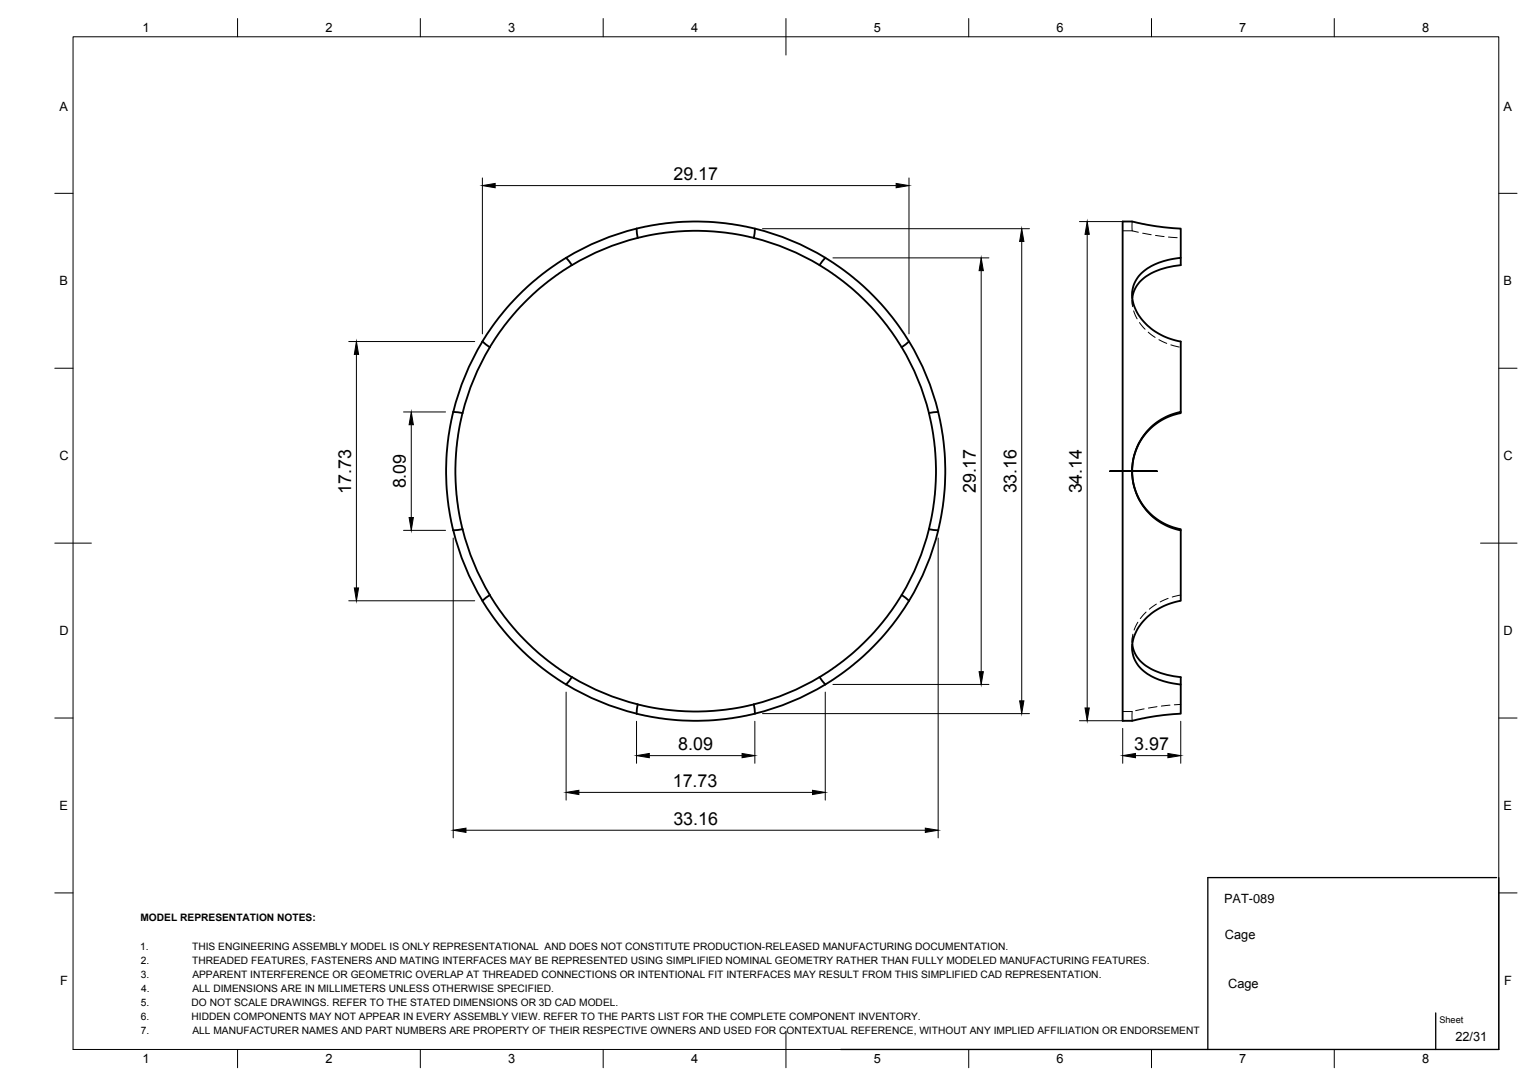
ISO-10303-21;
HEADER;
/* Generated by software containing ST-Developer
 * from STEP Tools, Inc. (www.steptools.com) 
 */

FILE_DESCRIPTION(
/* description */ ('Rotary union on bearing shaft'),
/* implementation_level */ '2;1');

FILE_NAME(
/* name */ 'Cage.step',
/* time_stamp */ '2026-10-28T03:24:01-07:00',
/* author */ (''),
/* organization */ (''),
/* preprocessor_version */ 'ST-DEVELOPER v20.2',
/* originating_system */ 'Autodesk Translation Framework v15.17.0.0',
/* authorisation */ '');

FILE_SCHEMA (('AUTOMOTIVE_DESIGN { 1 0 10303 214 3 1 1 }'));
ENDSEC;

DATA;
#10=MECHANICAL_DESIGN_GEOMETRIC_PRESENTATION_REPRESENTATION('',(#334),#9448);
#193=SPHERICAL_SURFACE('',#5486,0.412776);
#194=SPHERICAL_SURFACE('',#5502,0.412776);
#195=SPHERICAL_SURFACE('',#5507,0.412776);
#196=SPHERICAL_SURFACE('',#5512,0.412776);
#197=SPHERICAL_SURFACE('',#5517,0.412776);
#198=SPHERICAL_SURFACE('',#5522,0.412776);
#199=SPHERICAL_SURFACE('',#5527,0.412776);
#200=SPHERICAL_SURFACE('',#5535,0.412776);
#233=B_SPLINE_CURVE_WITH_KNOTS('',3,(#8136,#8137,#8138,#8139,#8140,#8141,
#8142,#8143,#8144,#8145,#8146,#8147,#8148,#8149,#8150,#8151,#8152,#8153,
#8154,#8155,#8156,#8157),.UNSPECIFIED.,.F.,.F.,(4,2,2,2,2,2,2,2,2,2,4),
(0.0789094028588958,0.210573405340968,0.315860108011452,0.421146810681936,
0.522142632548711,0.623138454415485,0.72413427628226,0.825130098149035,
0.930416800819519,1.03570350349,1.16736750597208),.UNSPECIFIED.);
#234=B_SPLINE_CURVE_WITH_KNOTS('',3,(#8161,#8162,#8163,#8164,#8165,#8166,
#8167,#8168,#8169,#8170,#8171,#8172,#8173,#8174,#8175,#8176,#8177,#8178,
#8179,#8180,#8181,#8182),.UNSPECIFIED.,.F.,.F.,(4,2,2,2,2,2,2,2,2,2,4),
(0.0774793363974613,0.142088896491891,0.284177792983782,0.411119756996526,
0.514392970548519,0.617666184100513,0.720939397652506,0.8242126112045,0.951154575217244,
1.09324347170913,1.15785303180356),.UNSPECIFIED.);
#235=B_SPLINE_CURVE_WITH_KNOTS('',3,(#8188,#8189,#8190,#8191,#8192,#8193,
#8194,#8195,#8196,#8197,#8198,#8199,#8200,#8201,#8202,#8203,#8204,#8205,
#8206,#8207,#8208,#8209),.UNSPECIFIED.,.F.,.F.,(4,2,2,2,2,2,2,2,2,2,4),
(0.0774793363974613,0.142088896491891,0.284177792983782,0.411119756996525,
0.514392970548519,0.617666184100513,0.720939397652506,0.8242126112045,0.951154575217243,
1.09324347170913,1.15785303180356),.UNSPECIFIED.);
#236=B_SPLINE_CURVE_WITH_KNOTS('',3,(#8213,#8214,#8215,#8216,#8217,#8218,
#8219,#8220,#8221,#8222,#8223,#8224,#8225,#8226,#8227,#8228,#8229,#8230,
#8231,#8232,#8233,#8234),.UNSPECIFIED.,.F.,.F.,(4,2,2,2,2,2,2,2,2,2,4),
(0.0774793363974614,0.142088896491891,0.284177792983781,0.411119756996525,
0.514392970548519,0.617666184100512,0.720939397652506,0.824212611204499,
0.951154575217243,1.09324347170913,1.15785303180356),.UNSPECIFIED.);
#237=B_SPLINE_CURVE_WITH_KNOTS('',3,(#8238,#8239,#8240,#8241,#8242,#8243,
#8244,#8245,#8246,#8247,#8248,#8249),.UNSPECIFIED.,.F.,.F.,(4,2,2,2,2,4),
(0.0774793363974613,0.142088896491891,0.284177792983781,0.411119756996525,
0.514392970548519,0.617666184100512),.UNSPECIFIED.);
#238=B_SPLINE_CURVE_WITH_KNOTS('',3,(#8254,#8255,#8256,#8257,#8258,#8259,
#8260,#8261,#8262,#8263,#8264,#8265),.UNSPECIFIED.,.F.,.F.,(4,2,2,2,2,4),
(0.617666184100512,0.720939397652506,0.824212611204499,0.951154575217243,
1.09324347170913,1.15785303180356),.UNSPECIFIED.);
#239=B_SPLINE_CURVE_WITH_KNOTS('',3,(#8269,#8270,#8271,#8272,#8273,#8274,
#8275,#8276,#8277,#8278,#8279,#8280,#8281,#8282,#8283,#8284,#8285,#8286,
#8287,#8288,#8289,#8290),.UNSPECIFIED.,.F.,.F.,(4,2,2,2,2,2,2,2,2,2,4),
(0.0774793363974613,0.142088896491891,0.284177792983782,0.411119756996526,
0.514392970548519,0.617666184100513,0.720939397652507,0.8242126112045,0.951154575217245,
1.09324347170914,1.15785303180356),.UNSPECIFIED.);
#240=B_SPLINE_CURVE_WITH_KNOTS('',3,(#8294,#8295,#8296,#8297,#8298,#8299,
#8300,#8301,#8302,#8303,#8304,#8305,#8306,#8307,#8308,#8309,#8310,#8311,
#8312,#8313,#8314,#8315),.UNSPECIFIED.,.F.,.F.,(4,2,2,2,2,2,2,2,2,2,4),
(0.0774793363974613,0.142088896491891,0.284177792983782,0.411119756996526,
0.514392970548519,0.617666184100513,0.720939397652506,0.824212611204499,
0.951154575217243,1.09324347170913,1.15785303180356),.UNSPECIFIED.);
#241=B_SPLINE_CURVE_WITH_KNOTS('',3,(#8319,#8320,#8321,#8322,#8323,#8324,
#8325,#8326,#8327,#8328,#8329,#8330,#8331,#8332,#8333,#8334,#8335,#8336,
#8337,#8338,#8339,#8340),.UNSPECIFIED.,.F.,.F.,(4,2,2,2,2,2,2,2,2,2,4),
(0.0774793363974613,0.142088896491891,0.284177792983782,0.411119756996526,
0.514392970548519,0.617666184100513,0.720939397652506,0.8242126112045,0.951154575217244,
1.09324347170913,1.15785303180356),.UNSPECIFIED.);
#242=B_SPLINE_CURVE_WITH_KNOTS('',3,(#8344,#8345,#8346,#8347,#8348,#8349,
#8350,#8351,#8352,#8353,#8354,#8355,#8356,#8357,#8358,#8359,#8360,#8361,
#8362,#8363,#8364,#8365),.UNSPECIFIED.,.F.,.F.,(4,2,2,2,2,2,2,2,2,2,4),
(0.0774793363974613,0.142088896491891,0.284177792983782,0.411119756996526,
0.514392970548519,0.617666184100513,0.720939397652506,0.8242126112045,0.951154575217243,
1.09324347170913,1.15785303180356),.UNSPECIFIED.);
#243=B_SPLINE_CURVE_WITH_KNOTS('',3,(#8373,#8374,#8375,#8376,#8377,#8378,
#8379,#8380,#8381,#8382,#8383,#8384,#8385,#8386,#8387,#8388,#8389,#8390,
#8391,#8392,#8393,#8394),.UNSPECIFIED.,.F.,.F.,(4,2,2,2,2,2,2,2,2,2,4),
(0.0789094028588958,0.210573405340968,0.315860108011452,0.421146810681936,
0.522142632548711,0.623138454415485,0.72413427628226,0.825130098149035,
0.930416800819519,1.03570350349,1.16736750597208),.UNSPECIFIED.);
#244=B_SPLINE_CURVE_WITH_KNOTS('',3,(#8402,#8403,#8404,#8405,#8406,#8407,
#8408,#8409,#8410,#8411,#8412,#8413,#8414,#8415,#8416,#8417,#8418,#8419,
#8420,#8421,#8422,#8423),.UNSPECIFIED.,.F.,.F.,(4,2,2,2,2,2,2,2,2,2,4),
(0.0789094028588958,0.210573405340969,0.315860108011453,0.421146810681937,
0.522142632548712,0.623138454415486,0.724134276282261,0.825130098149035,
0.930416800819519,1.03570350349,1.16736750597208),.UNSPECIFIED.);
#245=B_SPLINE_CURVE_WITH_KNOTS('',3,(#8432,#8433,#8434,#8435,#8436,#8437,
#8438,#8439,#8440,#8441,#8442,#8443),.UNSPECIFIED.,.F.,.F.,(4,2,2,2,2,4),
(0.0789094028588958,0.210573405340968,0.315860108011452,0.421146810681937,
0.522142632548711,0.623138454415486),.UNSPECIFIED.);
#246=B_SPLINE_CURVE_WITH_KNOTS('',3,(#8445,#8446,#8447,#8448,#8449,#8450,
#8451,#8452,#8453,#8454,#8455,#8456),.UNSPECIFIED.,.F.,.F.,(4,2,2,2,2,4),
(0.623138454415486,0.72413427628226,0.825130098149035,0.930416800819519,
1.03570350349,1.16736750597208),.UNSPECIFIED.);
#247=B_SPLINE_CURVE_WITH_KNOTS('',3,(#8463,#8464,#8465,#8466,#8467,#8468,
#8469,#8470,#8471,#8472,#8473,#8474,#8475,#8476,#8477,#8478,#8479,#8480,
#8481,#8482,#8483,#8484),.UNSPECIFIED.,.F.,.F.,(4,2,2,2,2,2,2,2,2,2,4),
(0.0789094028588958,0.210573405340968,0.315860108011452,0.421146810681936,
0.522142632548711,0.623138454415486,0.72413427628226,0.825130098149035,
0.930416800819519,1.03570350349,1.16736750597208),.UNSPECIFIED.);
#248=B_SPLINE_CURVE_WITH_KNOTS('',3,(#8492,#8493,#8494,#8495,#8496,#8497,
#8498,#8499,#8500,#8501,#8502,#8503,#8504,#8505,#8506,#8507,#8508,#8509,
#8510,#8511,#8512,#8513),.UNSPECIFIED.,.F.,.F.,(4,2,2,2,2,2,2,2,2,2,4),
(0.0789094028588957,0.210573405340968,0.315860108011452,0.421146810681936,
0.522142632548711,0.623138454415485,0.72413427628226,0.825130098149035,
0.930416800819519,1.03570350349,1.16736750597207),.UNSPECIFIED.);
#249=B_SPLINE_CURVE_WITH_KNOTS('',3,(#8521,#8522,#8523,#8524,#8525,#8526,
#8527,#8528,#8529,#8530,#8531,#8532,#8533,#8534,#8535,#8536,#8537,#8538,
#8539,#8540,#8541,#8542),.UNSPECIFIED.,.F.,.F.,(4,2,2,2,2,2,2,2,2,2,4),
(0.0789094028588958,0.210573405340968,0.315860108011452,0.421146810681936,
0.522142632548711,0.623138454415486,0.72413427628226,0.825130098149035,
0.930416800819519,1.03570350349,1.16736750597208),.UNSPECIFIED.);
#250=B_SPLINE_CURVE_WITH_KNOTS('',3,(#8551,#8552,#8553,#8554,#8555,#8556,
#8557,#8558,#8559,#8560,#8561,#8562,#8563,#8564,#8565,#8566,#8567,#8568,
#8569,#8570,#8571,#8572),.UNSPECIFIED.,.F.,.F.,(4,2,2,2,2,2,2,2,2,2,4),
(0.0789094028588958,0.210573405340968,0.315860108011452,0.421146810681936,
0.522142632548711,0.623138454415485,0.72413427628226,0.825130098149035,
0.930416800819519,1.03570350349,1.16736750597208),.UNSPECIFIED.);
#273=SHAPE_REPRESENTATION_RELATIONSHIP('SRR','None',#9574,#300);
#300=ADVANCED_BREP_SHAPE_REPRESENTATION('',(#369),#9434);
#334=STYLED_ITEM('',(#9778),#369);
#369=MANIFOLD_SOLID_BREP('Continuous crown cage',#4889);
#448=FACE_BOUND('',#1176,.T.);
#554=PLANE('',#5499);
#555=PLANE('',#5504);
#556=PLANE('',#5509);
#557=PLANE('',#5514);
#558=PLANE('',#5519);
#559=PLANE('',#5524);
#560=PLANE('',#5533);
#561=PLANE('',#5537);
#562=PLANE('',#5538);
#791=FACE_OUTER_BOUND('',#1158,.T.);
#792=FACE_OUTER_BOUND('',#1159,.T.);
#793=FACE_OUTER_BOUND('',#1160,.T.);
#794=FACE_OUTER_BOUND('',#1161,.T.);
#795=FACE_OUTER_BOUND('',#1162,.T.);
#796=FACE_OUTER_BOUND('',#1163,.T.);
#797=FACE_OUTER_BOUND('',#1164,.T.);
#798=FACE_OUTER_BOUND('',#1165,.T.);
#799=FACE_OUTER_BOUND('',#1166,.T.);
#800=FACE_OUTER_BOUND('',#1167,.T.);
#801=FACE_OUTER_BOUND('',#1168,.T.);
#802=FACE_OUTER_BOUND('',#1169,.T.);
#803=FACE_OUTER_BOUND('',#1170,.T.);
#804=FACE_OUTER_BOUND('',#1171,.T.);
#805=FACE_OUTER_BOUND('',#1172,.T.);
#806=FACE_OUTER_BOUND('',#1173,.T.);
#807=FACE_OUTER_BOUND('',#1174,.T.);
#808=FACE_OUTER_BOUND('',#1175,.T.);
#809=FACE_OUTER_BOUND('',#1177,.T.);
#1158=EDGE_LOOP('',(#3803,#3804,#3805,#3806));
#1159=EDGE_LOOP('',(#3807,#3808,#3809,#3810,#3811,#3812,#3813,#3814,#3815,
#3816,#3817,#3818,#3819,#3820,#3821,#3822,#3823,#3824,#3825,#3826));
#1160=EDGE_LOOP('',(#3827,#3828,#3829,#3830));
#1161=EDGE_LOOP('',(#3831,#3832,#3833,#3834));
#1162=EDGE_LOOP('',(#3835,#3836,#3837,#3838));
#1163=EDGE_LOOP('',(#3839,#3840,#3841,#3842));
#1164=EDGE_LOOP('',(#3843,#3844,#3845,#3846));
#1165=EDGE_LOOP('',(#3847,#3848,#3849,#3850,#3851,#3852));
#1166=EDGE_LOOP('',(#3853,#3854,#3855,#3856));
#1167=EDGE_LOOP('',(#3857,#3858,#3859,#3860));
#1168=EDGE_LOOP('',(#3861,#3862,#3863,#3864));
#1169=EDGE_LOOP('',(#3865,#3866,#3867,#3868));
#1170=EDGE_LOOP('',(#3869,#3870,#3871,#3872));
#1171=EDGE_LOOP('',(#3873,#3874,#3875,#3876));
#1172=EDGE_LOOP('',(#3877,#3878,#3879,#3880,#3881,#3882,#3883,#3884,#3885,
#3886,#3887,#3888,#3889,#3890,#3891,#3892,#3893,#3894,#3895,#3896));
#1173=EDGE_LOOP('',(#3897,#3898,#3899,#3900));
#1174=EDGE_LOOP('',(#3901,#3902,#3903,#3904));
#1175=EDGE_LOOP('',(#3905));
#1176=EDGE_LOOP('',(#3906));
#1177=EDGE_LOOP('',(#3907,#3908,#3909,#3910));
#1492=LINE('',#8251,#1812);
#1493=LINE('',#8547,#1813);
#1812=VECTOR('',#6537,1.706752);
#1813=VECTOR('',#6614,1.643248);
#2130=CIRCLE('',#5487,0.405071403305639);
#2131=CIRCLE('',#5488,0.405071403305639);
#2132=CIRCLE('',#5490,1.706752);
#2133=CIRCLE('',#5491,1.706752);
#2134=CIRCLE('',#5492,1.706752);
#2135=CIRCLE('',#5493,1.706752);
#2136=CIRCLE('',#5494,1.706752);
#2137=CIRCLE('',#5495,1.706752);
#2138=CIRCLE('',#5496,1.706752);
#2139=CIRCLE('',#5497,1.706752);
#2140=CIRCLE('',#5498,1.706752);
#2141=CIRCLE('',#5500,1.643248);
#2142=CIRCLE('',#5501,0.405071403305639);
#2143=CIRCLE('',#5503,0.405071403305639);
#2144=CIRCLE('',#5505,1.643248);
#2145=CIRCLE('',#5506,0.405071403305639);
#2146=CIRCLE('',#5508,0.405071403305639);
#2147=CIRCLE('',#5510,1.643248);
#2148=CIRCLE('',#5511,0.405071403305639);
#2149=CIRCLE('',#5513,0.405071403305639);
#2150=CIRCLE('',#5515,1.643248);
#2151=CIRCLE('',#5516,0.405071403305639);
#2152=CIRCLE('',#5518,0.405071403305639);
#2153=CIRCLE('',#5520,1.643248);
#2154=CIRCLE('',#5521,0.405071403305639);
#2155=CIRCLE('',#5523,0.405071403305639);
#2156=CIRCLE('',#5525,1.643248);
#2157=CIRCLE('',#5526,0.405071403305639);
#2158=CIRCLE('',#5528,0.405071403305639);
#2159=CIRCLE('',#5530,1.643248);
#2160=CIRCLE('',#5531,1.643248);
#2161=CIRCLE('',#5532,1.643248);
#2162=CIRCLE('',#5534,0.405071403305639);
#2163=CIRCLE('',#5536,0.405071403305639);
#2440=VERTEX_POINT('',#8134);
#2441=VERTEX_POINT('',#8135);
#2442=VERTEX_POINT('',#8158);
#2443=VERTEX_POINT('',#8160);
#2444=VERTEX_POINT('',#8185);
#2445=VERTEX_POINT('',#8187);
#2446=VERTEX_POINT('',#8210);
#2447=VERTEX_POINT('',#8212);
#2448=VERTEX_POINT('',#8235);
#2449=VERTEX_POINT('',#8237);
#2450=VERTEX_POINT('',#8250);
#2451=VERTEX_POINT('',#8253);
#2452=VERTEX_POINT('',#8266);
#2453=VERTEX_POINT('',#8268);
#2454=VERTEX_POINT('',#8291);
#2455=VERTEX_POINT('',#8293);
#2456=VERTEX_POINT('',#8316);
#2457=VERTEX_POINT('',#8318);
#2458=VERTEX_POINT('',#8341);
#2459=VERTEX_POINT('',#8343);
#2460=VERTEX_POINT('',#8368);
#2461=VERTEX_POINT('',#8372);
#2462=VERTEX_POINT('',#8397);
#2463=VERTEX_POINT('',#8401);
#2464=VERTEX_POINT('',#8426);
#2465=VERTEX_POINT('',#8430);
#2466=VERTEX_POINT('',#8431);
#2467=VERTEX_POINT('',#8458);
#2468=VERTEX_POINT('',#8462);
#2469=VERTEX_POINT('',#8487);
#2470=VERTEX_POINT('',#8491);
#2471=VERTEX_POINT('',#8516);
#2472=VERTEX_POINT('',#8520);
#2473=VERTEX_POINT('',#8545);
#2474=VERTEX_POINT('',#8548);
#2475=VERTEX_POINT('',#8550);
#2929=EDGE_CURVE('',#2440,#2441,#233,.T.);
#2930=EDGE_CURVE('',#2442,#2440,#2130,.T.);
#2931=EDGE_CURVE('',#2443,#2442,#234,.T.);
#2932=EDGE_CURVE('',#2441,#2443,#2131,.T.);
#2933=EDGE_CURVE('',#2444,#2442,#2132,.T.);
#2934=EDGE_CURVE('',#2444,#2445,#235,.T.);
#2935=EDGE_CURVE('',#2446,#2445,#2133,.T.);
#2936=EDGE_CURVE('',#2446,#2447,#236,.T.);
#2937=EDGE_CURVE('',#2448,#2447,#2134,.T.);
#2938=EDGE_CURVE('',#2448,#2449,#237,.T.);
#2939=EDGE_CURVE('',#2449,#2450,#1492,.T.);
#2940=EDGE_CURVE('',#2450,#2450,#2135,.T.);
#2941=EDGE_CURVE('',#2449,#2451,#238,.T.);
#2942=EDGE_CURVE('',#2452,#2451,#2136,.T.);
#2943=EDGE_CURVE('',#2452,#2453,#239,.T.);
#2944=EDGE_CURVE('',#2454,#2453,#2137,.T.);
#2945=EDGE_CURVE('',#2454,#2455,#240,.T.);
#2946=EDGE_CURVE('',#2456,#2455,#2138,.T.);
#2947=EDGE_CURVE('',#2456,#2457,#241,.T.);
#2948=EDGE_CURVE('',#2458,#2457,#2139,.T.);
#2949=EDGE_CURVE('',#2458,#2459,#242,.T.);
#2950=EDGE_CURVE('',#2443,#2459,#2140,.T.);
#2951=EDGE_CURVE('',#2440,#2460,#2141,.T.);
#2952=EDGE_CURVE('',#2460,#2444,#2142,.T.);
#2953=EDGE_CURVE('',#2461,#2460,#243,.T.);
#2954=EDGE_CURVE('',#2445,#2461,#2143,.T.);
#2955=EDGE_CURVE('',#2461,#2462,#2144,.T.);
#2956=EDGE_CURVE('',#2462,#2446,#2145,.T.);
#2957=EDGE_CURVE('',#2463,#2462,#244,.T.);
#2958=EDGE_CURVE('',#2447,#2463,#2146,.T.);
#2959=EDGE_CURVE('',#2463,#2464,#2147,.T.);
#2960=EDGE_CURVE('',#2464,#2448,#2148,.T.);
#2961=EDGE_CURVE('',#2465,#2466,#245,.T.);
#2962=EDGE_CURVE('',#2451,#2465,#2149,.T.);
#2963=EDGE_CURVE('',#2466,#2464,#246,.T.);
#2964=EDGE_CURVE('',#2465,#2467,#2150,.T.);
#2965=EDGE_CURVE('',#2467,#2452,#2151,.T.);
#2966=EDGE_CURVE('',#2468,#2467,#247,.T.);
#2967=EDGE_CURVE('',#2453,#2468,#2152,.T.);
#2968=EDGE_CURVE('',#2468,#2469,#2153,.T.);
#2969=EDGE_CURVE('',#2469,#2454,#2154,.T.);
#2970=EDGE_CURVE('',#2470,#2469,#248,.T.);
#2971=EDGE_CURVE('',#2455,#2470,#2155,.T.);
#2972=EDGE_CURVE('',#2470,#2471,#2156,.T.);
#2973=EDGE_CURVE('',#2471,#2456,#2157,.T.);
#2974=EDGE_CURVE('',#2472,#2471,#249,.T.);
#2975=EDGE_CURVE('',#2457,#2472,#2158,.T.);
#2976=EDGE_CURVE('',#2473,#2473,#2159,.T.);
#2977=EDGE_CURVE('',#2473,#2466,#1493,.T.);
#2978=EDGE_CURVE('',#2474,#2441,#2160,.T.);
#2979=EDGE_CURVE('',#2474,#2475,#250,.T.);
#2980=EDGE_CURVE('',#2472,#2475,#2161,.T.);
#2981=EDGE_CURVE('',#2459,#2474,#2162,.T.);
#2982=EDGE_CURVE('',#2475,#2458,#2163,.T.);
#3803=ORIENTED_EDGE('',*,*,#2929,.F.);
#3804=ORIENTED_EDGE('',*,*,#2930,.F.);
#3805=ORIENTED_EDGE('',*,*,#2931,.F.);
#3806=ORIENTED_EDGE('',*,*,#2932,.F.);
#3807=ORIENTED_EDGE('',*,*,#2931,.T.);
#3808=ORIENTED_EDGE('',*,*,#2933,.F.);
#3809=ORIENTED_EDGE('',*,*,#2934,.T.);
#3810=ORIENTED_EDGE('',*,*,#2935,.F.);
#3811=ORIENTED_EDGE('',*,*,#2936,.T.);
#3812=ORIENTED_EDGE('',*,*,#2937,.F.);
#3813=ORIENTED_EDGE('',*,*,#2938,.T.);
#3814=ORIENTED_EDGE('',*,*,#2939,.T.);
#3815=ORIENTED_EDGE('',*,*,#2940,.F.);
#3816=ORIENTED_EDGE('',*,*,#2939,.F.);
#3817=ORIENTED_EDGE('',*,*,#2941,.T.);
#3818=ORIENTED_EDGE('',*,*,#2942,.F.);
#3819=ORIENTED_EDGE('',*,*,#2943,.T.);
#3820=ORIENTED_EDGE('',*,*,#2944,.F.);
#3821=ORIENTED_EDGE('',*,*,#2945,.T.);
#3822=ORIENTED_EDGE('',*,*,#2946,.F.);
#3823=ORIENTED_EDGE('',*,*,#2947,.T.);
#3824=ORIENTED_EDGE('',*,*,#2948,.F.);
#3825=ORIENTED_EDGE('',*,*,#2949,.T.);
#3826=ORIENTED_EDGE('',*,*,#2950,.F.);
#3827=ORIENTED_EDGE('',*,*,#2930,.T.);
#3828=ORIENTED_EDGE('',*,*,#2951,.T.);
#3829=ORIENTED_EDGE('',*,*,#2952,.T.);
#3830=ORIENTED_EDGE('',*,*,#2933,.T.);
#3831=ORIENTED_EDGE('',*,*,#2953,.F.);
#3832=ORIENTED_EDGE('',*,*,#2954,.F.);
#3833=ORIENTED_EDGE('',*,*,#2934,.F.);
#3834=ORIENTED_EDGE('',*,*,#2952,.F.);
#3835=ORIENTED_EDGE('',*,*,#2954,.T.);
#3836=ORIENTED_EDGE('',*,*,#2955,.T.);
#3837=ORIENTED_EDGE('',*,*,#2956,.T.);
#3838=ORIENTED_EDGE('',*,*,#2935,.T.);
#3839=ORIENTED_EDGE('',*,*,#2957,.F.);
#3840=ORIENTED_EDGE('',*,*,#2958,.F.);
#3841=ORIENTED_EDGE('',*,*,#2936,.F.);
#3842=ORIENTED_EDGE('',*,*,#2956,.F.);
#3843=ORIENTED_EDGE('',*,*,#2958,.T.);
#3844=ORIENTED_EDGE('',*,*,#2959,.T.);
#3845=ORIENTED_EDGE('',*,*,#2960,.T.);
#3846=ORIENTED_EDGE('',*,*,#2937,.T.);
#3847=ORIENTED_EDGE('',*,*,#2961,.F.);
#3848=ORIENTED_EDGE('',*,*,#2962,.F.);
#3849=ORIENTED_EDGE('',*,*,#2941,.F.);
#3850=ORIENTED_EDGE('',*,*,#2938,.F.);
#3851=ORIENTED_EDGE('',*,*,#2960,.F.);
#3852=ORIENTED_EDGE('',*,*,#2963,.F.);
#3853=ORIENTED_EDGE('',*,*,#2962,.T.);
#3854=ORIENTED_EDGE('',*,*,#2964,.T.);
#3855=ORIENTED_EDGE('',*,*,#2965,.T.);
#3856=ORIENTED_EDGE('',*,*,#2942,.T.);
#3857=ORIENTED_EDGE('',*,*,#2966,.F.);
#3858=ORIENTED_EDGE('',*,*,#2967,.F.);
#3859=ORIENTED_EDGE('',*,*,#2943,.F.);
#3860=ORIENTED_EDGE('',*,*,#2965,.F.);
#3861=ORIENTED_EDGE('',*,*,#2967,.T.);
#3862=ORIENTED_EDGE('',*,*,#2968,.T.);
#3863=ORIENTED_EDGE('',*,*,#2969,.T.);
#3864=ORIENTED_EDGE('',*,*,#2944,.T.);
#3865=ORIENTED_EDGE('',*,*,#2970,.F.);
#3866=ORIENTED_EDGE('',*,*,#2971,.F.);
#3867=ORIENTED_EDGE('',*,*,#2945,.F.);
#3868=ORIENTED_EDGE('',*,*,#2969,.F.);
#3869=ORIENTED_EDGE('',*,*,#2971,.T.);
#3870=ORIENTED_EDGE('',*,*,#2972,.T.);
#3871=ORIENTED_EDGE('',*,*,#2973,.T.);
#3872=ORIENTED_EDGE('',*,*,#2946,.T.);
#3873=ORIENTED_EDGE('',*,*,#2947,.F.);
#3874=ORIENTED_EDGE('',*,*,#2973,.F.);
#3875=ORIENTED_EDGE('',*,*,#2974,.F.);
#3876=ORIENTED_EDGE('',*,*,#2975,.F.);
#3877=ORIENTED_EDGE('',*,*,#2976,.F.);
#3878=ORIENTED_EDGE('',*,*,#2977,.T.);
#3879=ORIENTED_EDGE('',*,*,#2963,.T.);
#3880=ORIENTED_EDGE('',*,*,#2959,.F.);
#3881=ORIENTED_EDGE('',*,*,#2957,.T.);
#3882=ORIENTED_EDGE('',*,*,#2955,.F.);
#3883=ORIENTED_EDGE('',*,*,#2953,.T.);
#3884=ORIENTED_EDGE('',*,*,#2951,.F.);
#3885=ORIENTED_EDGE('',*,*,#2929,.T.);
#3886=ORIENTED_EDGE('',*,*,#2978,.F.);
#3887=ORIENTED_EDGE('',*,*,#2979,.T.);
#3888=ORIENTED_EDGE('',*,*,#2980,.F.);
#3889=ORIENTED_EDGE('',*,*,#2974,.T.);
#3890=ORIENTED_EDGE('',*,*,#2972,.F.);
#3891=ORIENTED_EDGE('',*,*,#2970,.T.);
#3892=ORIENTED_EDGE('',*,*,#2968,.F.);
#3893=ORIENTED_EDGE('',*,*,#2966,.T.);
#3894=ORIENTED_EDGE('',*,*,#2964,.F.);
#3895=ORIENTED_EDGE('',*,*,#2961,.T.);
#3896=ORIENTED_EDGE('',*,*,#2977,.F.);
#3897=ORIENTED_EDGE('',*,*,#2932,.T.);
#3898=ORIENTED_EDGE('',*,*,#2950,.T.);
#3899=ORIENTED_EDGE('',*,*,#2981,.T.);
#3900=ORIENTED_EDGE('',*,*,#2978,.T.);
#3901=ORIENTED_EDGE('',*,*,#2949,.F.);
#3902=ORIENTED_EDGE('',*,*,#2982,.F.);
#3903=ORIENTED_EDGE('',*,*,#2979,.F.);
#3904=ORIENTED_EDGE('',*,*,#2981,.F.);
#3905=ORIENTED_EDGE('',*,*,#2940,.T.);
#3906=ORIENTED_EDGE('',*,*,#2976,.T.);
#3907=ORIENTED_EDGE('',*,*,#2975,.T.);
#3908=ORIENTED_EDGE('',*,*,#2980,.T.);
#3909=ORIENTED_EDGE('',*,*,#2982,.T.);
#3910=ORIENTED_EDGE('',*,*,#2948,.T.);
#4531=CYLINDRICAL_SURFACE('',#5489,1.706752);
#4532=CYLINDRICAL_SURFACE('',#5529,1.643248);
#4704=ADVANCED_FACE('',(#791),#193,.F.);
#4705=ADVANCED_FACE('',(#792),#4531,.T.);
#4706=ADVANCED_FACE('',(#793),#554,.T.);
#4707=ADVANCED_FACE('',(#794),#194,.F.);
#4708=ADVANCED_FACE('',(#795),#555,.T.);
#4709=ADVANCED_FACE('',(#796),#195,.F.);
#4710=ADVANCED_FACE('',(#797),#556,.T.);
#4711=ADVANCED_FACE('',(#798),#196,.F.);
#4712=ADVANCED_FACE('',(#799),#557,.T.);
#4713=ADVANCED_FACE('',(#800),#197,.F.);
#4714=ADVANCED_FACE('',(#801),#558,.T.);
#4715=ADVANCED_FACE('',(#802),#198,.F.);
#4716=ADVANCED_FACE('',(#803),#559,.T.);
#4717=ADVANCED_FACE('',(#804),#199,.F.);
#4718=ADVANCED_FACE('',(#805),#4532,.F.);
#4719=ADVANCED_FACE('',(#806),#560,.T.);
#4720=ADVANCED_FACE('',(#807),#200,.F.);
#4721=ADVANCED_FACE('',(#808,#448),#561,.T.);
#4722=ADVANCED_FACE('',(#809),#562,.T.);
#4889=CLOSED_SHELL('',(#4704,#4705,#4706,#4707,#4708,#4709,#4710,#4711,
#4712,#4713,#4714,#4715,#4716,#4717,#4718,#4719,#4720,#4721,#4722));
#5485=AXIS2_PLACEMENT_3D('',#8132,#6521,#6522);
#5486=AXIS2_PLACEMENT_3D('',#8133,#6523,#6524);
#5487=AXIS2_PLACEMENT_3D('',#8159,#6525,#6526);
#5488=AXIS2_PLACEMENT_3D('',#8183,#6527,#6528);
#5489=AXIS2_PLACEMENT_3D('',#8184,#6529,#6530);
#5490=AXIS2_PLACEMENT_3D('',#8186,#6531,#6532);
#5491=AXIS2_PLACEMENT_3D('',#8211,#6533,#6534);
#5492=AXIS2_PLACEMENT_3D('',#8236,#6535,#6536);
#5493=AXIS2_PLACEMENT_3D('',#8252,#6538,#6539);
#5494=AXIS2_PLACEMENT_3D('',#8267,#6540,#6541);
#5495=AXIS2_PLACEMENT_3D('',#8292,#6542,#6543);
#5496=AXIS2_PLACEMENT_3D('',#8317,#6544,#6545);
#5497=AXIS2_PLACEMENT_3D('',#8342,#6546,#6547);
#5498=AXIS2_PLACEMENT_3D('',#8366,#6548,#6549);
#5499=AXIS2_PLACEMENT_3D('',#8367,#6550,#6551);
#5500=AXIS2_PLACEMENT_3D('',#8369,#6552,#6553);
#5501=AXIS2_PLACEMENT_3D('',#8370,#6554,#6555);
#5502=AXIS2_PLACEMENT_3D('',#8371,#6556,#6557);
#5503=AXIS2_PLACEMENT_3D('',#8395,#6558,#6559);
#5504=AXIS2_PLACEMENT_3D('',#8396,#6560,#6561);
#5505=AXIS2_PLACEMENT_3D('',#8398,#6562,#6563);
#5506=AXIS2_PLACEMENT_3D('',#8399,#6564,#6565);
#5507=AXIS2_PLACEMENT_3D('',#8400,#6566,#6567);
#5508=AXIS2_PLACEMENT_3D('',#8424,#6568,#6569);
#5509=AXIS2_PLACEMENT_3D('',#8425,#6570,#6571);
#5510=AXIS2_PLACEMENT_3D('',#8427,#6572,#6573);
#5511=AXIS2_PLACEMENT_3D('',#8428,#6574,#6575);
#5512=AXIS2_PLACEMENT_3D('',#8429,#6576,#6577);
#5513=AXIS2_PLACEMENT_3D('',#8444,#6578,#6579);
#5514=AXIS2_PLACEMENT_3D('',#8457,#6580,#6581);
#5515=AXIS2_PLACEMENT_3D('',#8459,#6582,#6583);
#5516=AXIS2_PLACEMENT_3D('',#8460,#6584,#6585);
#5517=AXIS2_PLACEMENT_3D('',#8461,#6586,#6587);
#5518=AXIS2_PLACEMENT_3D('',#8485,#6588,#6589);
#5519=AXIS2_PLACEMENT_3D('',#8486,#6590,#6591);
#5520=AXIS2_PLACEMENT_3D('',#8488,#6592,#6593);
#5521=AXIS2_PLACEMENT_3D('',#8489,#6594,#6595);
#5522=AXIS2_PLACEMENT_3D('',#8490,#6596,#6597);
#5523=AXIS2_PLACEMENT_3D('',#8514,#6598,#6599);
#5524=AXIS2_PLACEMENT_3D('',#8515,#6600,#6601);
#5525=AXIS2_PLACEMENT_3D('',#8517,#6602,#6603);
#5526=AXIS2_PLACEMENT_3D('',#8518,#6604,#6605);
#5527=AXIS2_PLACEMENT_3D('',#8519,#6606,#6607);
#5528=AXIS2_PLACEMENT_3D('',#8543,#6608,#6609);
#5529=AXIS2_PLACEMENT_3D('',#8544,#6610,#6611);
#5530=AXIS2_PLACEMENT_3D('',#8546,#6612,#6613);
#5531=AXIS2_PLACEMENT_3D('',#8549,#6615,#6616);
#5532=AXIS2_PLACEMENT_3D('',#8573,#6617,#6618);
#5533=AXIS2_PLACEMENT_3D('',#8574,#6619,#6620);
#5534=AXIS2_PLACEMENT_3D('',#8575,#6621,#6622);
#5535=AXIS2_PLACEMENT_3D('',#8576,#6623,#6624);
#5536=AXIS2_PLACEMENT_3D('',#8577,#6625,#6626);
#5537=AXIS2_PLACEMENT_3D('',#8578,#6627,#6628);
#5538=AXIS2_PLACEMENT_3D('',#8579,#6629,#6630);
#6521=DIRECTION('axis',(0.,0.,1.));
#6522=DIRECTION('refdir',(1.,0.,0.));
#6523=DIRECTION('center_axis',(0.,0.,1.));
#6524=DIRECTION('ref_axis',(1.,0.,0.));
#6525=DIRECTION('center_axis',(0.,-1.,0.));
#6526=DIRECTION('ref_axis',(0.,0.,-1.));
#6527=DIRECTION('center_axis',(0.,-1.,0.));
#6528=DIRECTION('ref_axis',(0.,0.,-1.));
#6529=DIRECTION('center_axis',(0.,1.,0.));
#6530=DIRECTION('ref_axis',(1.,0.,0.));
#6531=DIRECTION('center_axis',(0.,1.,0.));
#6532=DIRECTION('ref_axis',(1.,0.,0.));
#6533=DIRECTION('center_axis',(0.,1.,0.));
#6534=DIRECTION('ref_axis',(1.,0.,0.));
#6535=DIRECTION('center_axis',(0.,1.,0.));
#6536=DIRECTION('ref_axis',(1.,0.,0.));
#6537=DIRECTION('',(0.,-1.,0.));
#6538=DIRECTION('center_axis',(0.,-1.,0.));
#6539=DIRECTION('ref_axis',(1.,0.,0.));
#6540=DIRECTION('center_axis',(0.,1.,0.));
#6541=DIRECTION('ref_axis',(1.,0.,0.));
#6542=DIRECTION('center_axis',(0.,1.,0.));
#6543=DIRECTION('ref_axis',(1.,0.,0.));
#6544=DIRECTION('center_axis',(0.,1.,0.));
#6545=DIRECTION('ref_axis',(1.,0.,0.));
#6546=DIRECTION('center_axis',(0.,1.,0.));
#6547=DIRECTION('ref_axis',(1.,0.,0.));
#6548=DIRECTION('center_axis',(0.,1.,0.));
#6549=DIRECTION('ref_axis',(1.,0.,0.));
#6550=DIRECTION('center_axis',(0.,1.,0.));
#6551=DIRECTION('ref_axis',(1.,0.,0.));
#6552=DIRECTION('center_axis',(0.,-1.,0.));
#6553=DIRECTION('ref_axis',(1.,0.,0.));
#6554=DIRECTION('center_axis',(0.,-1.,0.));
#6555=DIRECTION('ref_axis',(0.,0.,-1.));
#6556=DIRECTION('center_axis',(6.12323399573677E-17,0.,1.));
#6557=DIRECTION('ref_axis',(1.,0.,0.));
#6558=DIRECTION('center_axis',(0.,-1.,0.));
#6559=DIRECTION('ref_axis',(0.,0.,-1.));
#6560=DIRECTION('center_axis',(0.,1.,0.));
#6561=DIRECTION('ref_axis',(1.,0.,0.));
#6562=DIRECTION('center_axis',(0.,-1.,0.));
#6563=DIRECTION('ref_axis',(1.,0.,0.));
#6564=DIRECTION('center_axis',(0.,-1.,0.));
#6565=DIRECTION('ref_axis',(0.,0.,-1.));
#6566=DIRECTION('center_axis',(0.,0.,1.));
#6567=DIRECTION('ref_axis',(1.,0.,0.));
#6568=DIRECTION('center_axis',(0.,-1.,0.));
#6569=DIRECTION('ref_axis',(0.,0.,-1.));
#6570=DIRECTION('center_axis',(0.,1.,0.));
#6571=DIRECTION('ref_axis',(1.,0.,0.));
#6572=DIRECTION('center_axis',(0.,-1.,0.));
#6573=DIRECTION('ref_axis',(1.,0.,0.));
#6574=DIRECTION('center_axis',(0.,-1.,0.));
#6575=DIRECTION('ref_axis',(0.,0.,-1.));
#6576=DIRECTION('center_axis',(0.,0.,1.));
#6577=DIRECTION('ref_axis',(1.,0.,0.));
#6578=DIRECTION('center_axis',(0.,-1.,0.));
#6579=DIRECTION('ref_axis',(0.,0.,-1.));
#6580=DIRECTION('center_axis',(0.,1.,0.));
#6581=DIRECTION('ref_axis',(1.,0.,0.));
#6582=DIRECTION('center_axis',(0.,-1.,0.));
#6583=DIRECTION('ref_axis',(1.,0.,0.));
#6584=DIRECTION('center_axis',(0.,-1.,0.));
#6585=DIRECTION('ref_axis',(0.,0.,-1.));
#6586=DIRECTION('center_axis',(0.,0.,1.));
#6587=DIRECTION('ref_axis',(1.,0.,0.));
#6588=DIRECTION('center_axis',(0.,-1.,0.));
#6589=DIRECTION('ref_axis',(0.,0.,-1.));
#6590=DIRECTION('center_axis',(0.,1.,0.));
#6591=DIRECTION('ref_axis',(1.,0.,0.));
#6592=DIRECTION('center_axis',(0.,-1.,0.));
#6593=DIRECTION('ref_axis',(1.,0.,0.));
#6594=DIRECTION('center_axis',(0.,-1.,0.));
#6595=DIRECTION('ref_axis',(0.,0.,-1.));
#6596=DIRECTION('center_axis',(6.12323399573676E-17,0.,1.));
#6597=DIRECTION('ref_axis',(1.,0.,0.));
#6598=DIRECTION('center_axis',(0.,-1.,0.));
#6599=DIRECTION('ref_axis',(0.,0.,-1.));
#6600=DIRECTION('center_axis',(0.,1.,0.));
#6601=DIRECTION('ref_axis',(1.,0.,0.));
#6602=DIRECTION('center_axis',(0.,-1.,0.));
#6603=DIRECTION('ref_axis',(1.,0.,0.));
#6604=DIRECTION('center_axis',(0.,-1.,0.));
#6605=DIRECTION('ref_axis',(0.,0.,-1.));
#6606=DIRECTION('center_axis',(0.,0.,1.));
#6607=DIRECTION('ref_axis',(1.,0.,0.));
#6608=DIRECTION('center_axis',(0.,-1.,0.));
#6609=DIRECTION('ref_axis',(0.,0.,-1.));
#6610=DIRECTION('center_axis',(0.,1.,0.));
#6611=DIRECTION('ref_axis',(1.,0.,0.));
#6612=DIRECTION('center_axis',(0.,1.,0.));
#6613=DIRECTION('ref_axis',(1.,0.,0.));
#6614=DIRECTION('',(0.,1.,0.));
#6615=DIRECTION('center_axis',(0.,-1.,0.));
#6616=DIRECTION('ref_axis',(1.,0.,0.));
#6617=DIRECTION('center_axis',(0.,-1.,0.));
#6618=DIRECTION('ref_axis',(1.,0.,0.));
#6619=DIRECTION('center_axis',(0.,1.,0.));
#6620=DIRECTION('ref_axis',(1.,0.,0.));
#6621=DIRECTION('center_axis',(0.,-1.,0.));
#6622=DIRECTION('ref_axis',(0.,0.,-1.));
#6623=DIRECTION('center_axis',(0.,0.,1.));
#6624=DIRECTION('ref_axis',(1.,0.,0.));
#6625=DIRECTION('center_axis',(0.,-1.,0.));
#6626=DIRECTION('ref_axis',(0.,0.,-1.));
#6627=DIRECTION('center_axis',(0.,-1.,0.));
#6628=DIRECTION('ref_axis',(-1.,0.,0.));
#6629=DIRECTION('center_axis',(0.,1.,0.));
#6630=DIRECTION('ref_axis',(1.,0.,0.));
#8132=CARTESIAN_POINT('',(0.,0.,0.));
#8133=CARTESIAN_POINT('Origin',(1.18440385848747,0.,1.18440385848747));
#8134=CARTESIAN_POINT('',(0.846804978391753,-0.07938,1.40825612658882));
#8135=CARTESIAN_POINT('',(1.40825612658882,-0.07938,0.846804978391754));
#8136=CARTESIAN_POINT('Ctrl Pts',(0.846804978391752,-0.0793800000000001,
1.40825612658882));
#8137=CARTESIAN_POINT('Ctrl Pts',(0.854205272175554,-0.123401821157026,
1.40380622184538));
#8138=CARTESIAN_POINT('Ctrl Pts',(0.867957148219441,-0.166543350814306,
1.39550172959303));
#8139=CARTESIAN_POINT('Ctrl Pts',(0.902193646979982,-0.237231147975234,
1.3735491215176));
#8140=CARTESIAN_POINT('Ctrl Pts',(0.920778333482564,-0.266264900654909,
1.36127834356734));
#8141=CARTESIAN_POINT('Ctrl Pts',(0.962485392528369,-0.317195968905306,
1.33211611256184));
#8142=CARTESIAN_POINT('Ctrl Pts',(0.985600426557816,-0.33909093068465,1.31521005565926));
#8143=CARTESIAN_POINT('Ctrl Pts',(1.03253285680459,-0.373586846396559,1.27866649102984));
#8144=CARTESIAN_POINT('Ctrl Pts',(1.05871835910697,-0.388086240756494,1.25722555095714));
#8145=CARTESIAN_POINT('Ctrl Pts',(1.11153475808518,-0.407068917407805,1.2107812086231));
#8146=CARTESIAN_POINT('Ctrl Pts',(1.13814686046673,-0.411552957311693,1.18575674747573));
#8147=CARTESIAN_POINT('Ctrl Pts',(1.18575674747573,-0.411552957311693,1.13814686046673));
#8148=CARTESIAN_POINT('Ctrl Pts',(1.2107812086231,-0.407068917407805,1.11153475808518));
#8149=CARTESIAN_POINT('Ctrl Pts',(1.25722555095713,-0.388086240756494,1.05871835910697));
#8150=CARTESIAN_POINT('Ctrl Pts',(1.27866649102984,-0.373586846396559,1.03253285680459));
#8151=CARTESIAN_POINT('Ctrl Pts',(1.31521005565926,-0.33909093068465,0.985600426557816));
#8152=CARTESIAN_POINT('Ctrl Pts',(1.33211611256184,-0.317195968905306,0.962485392528369));
#8153=CARTESIAN_POINT('Ctrl Pts',(1.36127834356734,-0.266264900654909,0.920778333482565));
#8154=CARTESIAN_POINT('Ctrl Pts',(1.3735491215176,-0.237231147975234,0.902193646979983));
#8155=CARTESIAN_POINT('Ctrl Pts',(1.39550172959303,-0.166543350814306,0.867957148219442));
#8156=CARTESIAN_POINT('Ctrl Pts',(1.40380622184538,-0.123401821157026,0.854205272175555));
#8157=CARTESIAN_POINT('Ctrl Pts',(1.40825612658882,-0.0793800000000001,
0.846804978391753));
#8158=CARTESIAN_POINT('',(0.886256117232623,-0.07938,1.45861320581289));
#8159=CARTESIAN_POINT('Origin',(1.18440385848747,-0.07938,1.18440385848747));
#8160=CARTESIAN_POINT('',(1.45861320581289,-0.07938,0.886256117232624));
#8161=CARTESIAN_POINT('Ctrl Pts',(1.45861320581289,-0.0793800000000001,
0.886256117232623));
#8162=CARTESIAN_POINT('Ctrl Pts',(1.45630208793976,-0.101649918886749,0.890059788636852));
#8163=CARTESIAN_POINT('Ctrl Pts',(1.45296717977858,-0.123823518623746,0.895520212222107));
#8164=CARTESIAN_POINT('Ctrl Pts',(1.43904931717599,-0.192480977588836,0.917859913453975));
#8165=CARTESIAN_POINT('Ctrl Pts',(1.4243271592157,-0.236152929235938,0.940896403863072));
#8166=CARTESIAN_POINT('Ctrl Pts',(1.39055359345152,-0.303141259068212,0.990027513266106));
#8167=CARTESIAN_POINT('Ctrl Pts',(1.36743459453896,-0.335108247315849,1.02199477007745));
#8168=CARTESIAN_POINT('Ctrl Pts',(1.32643091652006,-0.373243761060364,1.07446535104584));
#8169=CARTESIAN_POINT('Ctrl Pts',(1.30441816675528,-0.387888272594439,1.10126842659597));
#8170=CARTESIAN_POINT('Ctrl Pts',(1.25681160160691,-0.407041111792943,1.15530234155453));
#8171=CARTESIAN_POINT('Ctrl Pts',(1.23119764287622,-0.411552957311693,1.18251418313119));
#8172=CARTESIAN_POINT('Ctrl Pts',(1.18251418313119,-0.411552957311693,1.23119764287622));
#8173=CARTESIAN_POINT('Ctrl Pts',(1.15530234155453,-0.407041111792943,1.25681160160691));
#8174=CARTESIAN_POINT('Ctrl Pts',(1.10126842659597,-0.387888272594439,1.30441816675528));
#8175=CARTESIAN_POINT('Ctrl Pts',(1.07446535104584,-0.373243761060364,1.32643091652006));
#8176=CARTESIAN_POINT('Ctrl Pts',(1.02199477007745,-0.335108247315848,1.36743459453896));
#8177=CARTESIAN_POINT('Ctrl Pts',(0.990027513266105,-0.303141259068211,
1.39055359345152));
#8178=CARTESIAN_POINT('Ctrl Pts',(0.940896403863071,-0.236152929235937,
1.42432715921571));
#8179=CARTESIAN_POINT('Ctrl Pts',(0.917859913453974,-0.192480977588835,
1.43904931717599));
#8180=CARTESIAN_POINT('Ctrl Pts',(0.895520212222106,-0.123823518623745,
1.45296717977858));
#8181=CARTESIAN_POINT('Ctrl Pts',(0.890059788636851,-0.101649918886749,
1.45630208793976));
#8182=CARTESIAN_POINT('Ctrl Pts',(0.886256117232622,-0.0793800000000001,
1.45861320581289));
#8183=CARTESIAN_POINT('Origin',(1.18440385848747,-0.07938,1.18440385848747));
#8184=CARTESIAN_POINT('Origin',(0.,-0.27783,0.));
#8185=CARTESIAN_POINT('',(0.404717578595295,-0.07938,1.65807299932179));
#8186=CARTESIAN_POINT('Origin',(0.,-0.07938,0.));
#8187=CARTESIAN_POINT('',(-0.404717578595296,-0.07938,1.65807299932179));
#8188=CARTESIAN_POINT('Ctrl Pts',(0.404717578595296,-0.0793800000000001,
1.65807299932179));
#8189=CARTESIAN_POINT('Ctrl Pts',(0.400393769631747,-0.101649918886749,
1.65912839404491));
#8190=CARTESIAN_POINT('Ctrl Pts',(0.394174530911058,-0.123823518623745,
1.66063136041479));
#8191=CARTESIAN_POINT('Ctrl Pts',(0.368536561654407,-0.192480977588835,
1.66658649961961));
#8192=CARTESIAN_POINT('Ctrl Pts',(0.341837165343982,-0.236152929235937,
1.67246562047521));
#8193=CARTESIAN_POINT('Ctrl Pts',(0.283214707341173,-0.303141259068211,
1.68332504372461));
#8194=CARTESIAN_POINT('Ctrl Pts',(0.244262842368623,-0.335108247315849,
1.68958170688653));
#8195=CARTESIAN_POINT('Ctrl Pts',(0.178166559972324,-0.373243761060364,
1.69769003172132));
#8196=CARTESIAN_POINT('Ctrl Pts',(0.143648558862931,-0.387888272594439,
1.70107730356824));
#8197=CARTESIAN_POINT('Ctrl Pts',(0.0717778861362652,-0.407041111792943,
1.70562212620408));
#8198=CARTESIAN_POINT('Ctrl Pts',(0.0344244045173309,-0.411552957311693,
1.706752));
#8199=CARTESIAN_POINT('Ctrl Pts',(-0.0344244045173315,-0.411552957311693,
1.706752));
#8200=CARTESIAN_POINT('Ctrl Pts',(-0.0717778861362658,-0.407041111792943,
1.70562212620408));
#8201=CARTESIAN_POINT('Ctrl Pts',(-0.143648558862932,-0.387888272594439,
1.70107730356824));
#8202=CARTESIAN_POINT('Ctrl Pts',(-0.178166559972325,-0.373243761060364,
1.69769003172132));
#8203=CARTESIAN_POINT('Ctrl Pts',(-0.244262842368624,-0.335108247315849,
1.68958170688653));
#8204=CARTESIAN_POINT('Ctrl Pts',(-0.283214707341173,-0.303141259068212,
1.68332504372461));
#8205=CARTESIAN_POINT('Ctrl Pts',(-0.341837165343982,-0.236152929235937,
1.67246562047521));
#8206=CARTESIAN_POINT('Ctrl Pts',(-0.368536561654408,-0.192480977588835,
1.66658649961961));
#8207=CARTESIAN_POINT('Ctrl Pts',(-0.394174530911059,-0.123823518623745,
1.66063136041479));
#8208=CARTESIAN_POINT('Ctrl Pts',(-0.400393769631748,-0.101649918886749,
1.65912839404491));
#8209=CARTESIAN_POINT('Ctrl Pts',(-0.404717578595297,-0.0793800000000001,
1.65807299932179));
#8210=CARTESIAN_POINT('',(-0.886256117232624,-0.07938,1.45861320581289));
#8211=CARTESIAN_POINT('Origin',(0.,-0.07938,0.));
#8212=CARTESIAN_POINT('',(-1.45861320581289,-0.07938,0.886256117232623));
#8213=CARTESIAN_POINT('Ctrl Pts',(-0.886256117232623,-0.0793800000000001,
1.45861320581289));
#8214=CARTESIAN_POINT('Ctrl Pts',(-0.890059788636852,-0.101649918886749,
1.45630208793976));
#8215=CARTESIAN_POINT('Ctrl Pts',(-0.895520212222106,-0.123823518623745,
1.45296717977858));
#8216=CARTESIAN_POINT('Ctrl Pts',(-0.917859913453974,-0.192480977588835,
1.43904931717599));
#8217=CARTESIAN_POINT('Ctrl Pts',(-0.940896403863071,-0.236152929235937,
1.4243271592157));
#8218=CARTESIAN_POINT('Ctrl Pts',(-0.990027513266105,-0.303141259068211,
1.39055359345152));
#8219=CARTESIAN_POINT('Ctrl Pts',(-1.02199477007745,-0.335108247315848,
1.36743459453896));
#8220=CARTESIAN_POINT('Ctrl Pts',(-1.07446535104584,-0.373243761060364,
1.32643091652006));
#8221=CARTESIAN_POINT('Ctrl Pts',(-1.10126842659597,-0.387888272594439,
1.30441816675528));
#8222=CARTESIAN_POINT('Ctrl Pts',(-1.15530234155453,-0.407041111792943,
1.25681160160691));
#8223=CARTESIAN_POINT('Ctrl Pts',(-1.18251418313119,-0.411552957311693,
1.23119764287622));
#8224=CARTESIAN_POINT('Ctrl Pts',(-1.23119764287622,-0.411552957311693,
1.18251418313119));
#8225=CARTESIAN_POINT('Ctrl Pts',(-1.25681160160691,-0.407041111792943,
1.15530234155453));
#8226=CARTESIAN_POINT('Ctrl Pts',(-1.30441816675528,-0.387888272594439,
1.10126842659597));
#8227=CARTESIAN_POINT('Ctrl Pts',(-1.32643091652006,-0.373243761060365,
1.07446535104584));
#8228=CARTESIAN_POINT('Ctrl Pts',(-1.36743459453896,-0.335108247315849,
1.02199477007745));
#8229=CARTESIAN_POINT('Ctrl Pts',(-1.39055359345152,-0.303141259068212,
0.990027513266106));
#8230=CARTESIAN_POINT('Ctrl Pts',(-1.4243271592157,-0.236152929235938,0.940896403863071));
#8231=CARTESIAN_POINT('Ctrl Pts',(-1.43904931717599,-0.192480977588836,
0.917859913453974));
#8232=CARTESIAN_POINT('Ctrl Pts',(-1.45296717977858,-0.123823518623746,
0.895520212222106));
#8233=CARTESIAN_POINT('Ctrl Pts',(-1.45630208793976,-0.101649918886749,
0.890059788636852));
#8234=CARTESIAN_POINT('Ctrl Pts',(-1.45861320581289,-0.0793800000000001,
0.886256117232623));
#8235=CARTESIAN_POINT('',(-1.65807299932179,-0.07938,0.404717578595295));
#8236=CARTESIAN_POINT('Origin',(0.,-0.07938,0.));
#8237=CARTESIAN_POINT('',(-1.706752,-0.411552957311693,2.08591827245526E-16));
#8238=CARTESIAN_POINT('Ctrl Pts',(-1.65807299932179,-0.0793800000000001,
0.404717578595296));
#8239=CARTESIAN_POINT('Ctrl Pts',(-1.65912839404491,-0.101649918886749,
0.400393769631747));
#8240=CARTESIAN_POINT('Ctrl Pts',(-1.66063136041479,-0.123823518623745,
0.394174530911058));
#8241=CARTESIAN_POINT('Ctrl Pts',(-1.66658649961961,-0.192480977588835,
0.368536561654407));
#8242=CARTESIAN_POINT('Ctrl Pts',(-1.67246562047521,-0.236152929235937,
0.341837165343982));
#8243=CARTESIAN_POINT('Ctrl Pts',(-1.68332504372461,-0.303141259068211,
0.283214707341173));
#8244=CARTESIAN_POINT('Ctrl Pts',(-1.68958170688653,-0.335108247315848,
0.244262842368623));
#8245=CARTESIAN_POINT('Ctrl Pts',(-1.69769003172132,-0.373243761060364,
0.178166559972324));
#8246=CARTESIAN_POINT('Ctrl Pts',(-1.70107730356824,-0.387888272594439,
0.143648558862931));
#8247=CARTESIAN_POINT('Ctrl Pts',(-1.70562212620408,-0.407041111792943,
0.0717778861362656));
#8248=CARTESIAN_POINT('Ctrl Pts',(-1.706752,-0.411552957311693,0.0344244045173313));
#8249=CARTESIAN_POINT('Ctrl Pts',(-1.706752,-0.411552957311693,2.08166817117217E-16));
#8250=CARTESIAN_POINT('',(-1.706752,-0.47628,2.09016837373834E-16));
#8251=CARTESIAN_POINT('',(-1.706752,-0.27783,2.09016837373834E-16));
#8252=CARTESIAN_POINT('Origin',(0.,-0.47628,0.));
#8253=CARTESIAN_POINT('',(-1.65807299932179,-0.07938,-0.404717578595296));
#8254=CARTESIAN_POINT('Ctrl Pts',(-1.706752,-0.411552957311693,2.0122792321331E-16));
#8255=CARTESIAN_POINT('Ctrl Pts',(-1.706752,-0.411552957311693,-0.0344244045173309));
#8256=CARTESIAN_POINT('Ctrl Pts',(-1.70562212620408,-0.407041111792943,
-0.0717778861362652));
#8257=CARTESIAN_POINT('Ctrl Pts',(-1.70107730356824,-0.387888272594439,
-0.143648558862931));
#8258=CARTESIAN_POINT('Ctrl Pts',(-1.69769003172132,-0.373243761060365,
-0.178166559972324));
#8259=CARTESIAN_POINT('Ctrl Pts',(-1.68958170688653,-0.335108247315849,
-0.244262842368623));
#8260=CARTESIAN_POINT('Ctrl Pts',(-1.68332504372461,-0.303141259068212,
-0.283214707341173));
#8261=CARTESIAN_POINT('Ctrl Pts',(-1.67246562047521,-0.236152929235938,
-0.341837165343982));
#8262=CARTESIAN_POINT('Ctrl Pts',(-1.66658649961961,-0.192480977588836,
-0.368536561654407));
#8263=CARTESIAN_POINT('Ctrl Pts',(-1.66063136041479,-0.123823518623745,
-0.394174530911059));
#8264=CARTESIAN_POINT('Ctrl Pts',(-1.65912839404491,-0.101649918886749,
-0.400393769631748));
#8265=CARTESIAN_POINT('Ctrl Pts',(-1.65807299932179,-0.0793800000000001,
-0.404717578595296));
#8266=CARTESIAN_POINT('',(-1.45861320581289,-0.07938,-0.886256117232623));
#8267=CARTESIAN_POINT('Origin',(0.,-0.07938,0.));
#8268=CARTESIAN_POINT('',(-0.886256117232623,-0.07938,-1.45861320581289));
#8269=CARTESIAN_POINT('Ctrl Pts',(-1.45861320581289,-0.0793800000000001,
-0.886256117232623));
#8270=CARTESIAN_POINT('Ctrl Pts',(-1.45630208793976,-0.101649918886749,
-0.890059788636852));
#8271=CARTESIAN_POINT('Ctrl Pts',(-1.45296717977858,-0.123823518623745,
-0.895520212222106));
#8272=CARTESIAN_POINT('Ctrl Pts',(-1.43904931717599,-0.192480977588835,
-0.917859913453974));
#8273=CARTESIAN_POINT('Ctrl Pts',(-1.4243271592157,-0.236152929235937,-0.940896403863072));
#8274=CARTESIAN_POINT('Ctrl Pts',(-1.39055359345152,-0.303141259068212,
-0.990027513266106));
#8275=CARTESIAN_POINT('Ctrl Pts',(-1.36743459453896,-0.335108247315849,
-1.02199477007745));
#8276=CARTESIAN_POINT('Ctrl Pts',(-1.32643091652006,-0.373243761060364,
-1.07446535104584));
#8277=CARTESIAN_POINT('Ctrl Pts',(-1.30441816675528,-0.387888272594439,
-1.10126842659597));
#8278=CARTESIAN_POINT('Ctrl Pts',(-1.25681160160691,-0.407041111792943,
-1.15530234155453));
#8279=CARTESIAN_POINT('Ctrl Pts',(-1.23119764287622,-0.411552957311693,
-1.18251418313119));
#8280=CARTESIAN_POINT('Ctrl Pts',(-1.18251418313119,-0.411552957311693,
-1.23119764287622));
#8281=CARTESIAN_POINT('Ctrl Pts',(-1.15530234155453,-0.407041111792943,
-1.25681160160691));
#8282=CARTESIAN_POINT('Ctrl Pts',(-1.10126842659597,-0.387888272594439,
-1.30441816675528));
#8283=CARTESIAN_POINT('Ctrl Pts',(-1.07446535104584,-0.373243761060364,
-1.32643091652006));
#8284=CARTESIAN_POINT('Ctrl Pts',(-1.02199477007745,-0.335108247315848,
-1.36743459453896));
#8285=CARTESIAN_POINT('Ctrl Pts',(-0.990027513266105,-0.303141259068211,
-1.39055359345152));
#8286=CARTESIAN_POINT('Ctrl Pts',(-0.940896403863071,-0.236152929235936,
-1.42432715921571));
#8287=CARTESIAN_POINT('Ctrl Pts',(-0.917859913453974,-0.192480977588835,
-1.43904931717599));
#8288=CARTESIAN_POINT('Ctrl Pts',(-0.895520212222106,-0.123823518623745,
-1.45296717977858));
#8289=CARTESIAN_POINT('Ctrl Pts',(-0.890059788636851,-0.101649918886749,
-1.45630208793976));
#8290=CARTESIAN_POINT('Ctrl Pts',(-0.886256117232623,-0.0793800000000001,
-1.45861320581289));
#8291=CARTESIAN_POINT('',(-0.404717578595295,-0.07938,-1.65807299932179));
#8292=CARTESIAN_POINT('Origin',(0.,-0.07938,0.));
#8293=CARTESIAN_POINT('',(0.404717578595296,-0.07938,-1.65807299932179));
#8294=CARTESIAN_POINT('Ctrl Pts',(-0.404717578595296,-0.0793800000000001,
-1.65807299932179));
#8295=CARTESIAN_POINT('Ctrl Pts',(-0.400393769631747,-0.101649918886749,
-1.65912839404491));
#8296=CARTESIAN_POINT('Ctrl Pts',(-0.394174530911058,-0.123823518623746,
-1.66063136041479));
#8297=CARTESIAN_POINT('Ctrl Pts',(-0.368536561654407,-0.192480977588836,
-1.66658649961961));
#8298=CARTESIAN_POINT('Ctrl Pts',(-0.341837165343982,-0.236152929235938,
-1.67246562047521));
#8299=CARTESIAN_POINT('Ctrl Pts',(-0.283214707341173,-0.303141259068212,
-1.68332504372461));
#8300=CARTESIAN_POINT('Ctrl Pts',(-0.244262842368623,-0.335108247315849,
-1.68958170688653));
#8301=CARTESIAN_POINT('Ctrl Pts',(-0.178166559972324,-0.373243761060364,
-1.69769003172132));
#8302=CARTESIAN_POINT('Ctrl Pts',(-0.143648558862931,-0.387888272594439,
-1.70107730356824));
#8303=CARTESIAN_POINT('Ctrl Pts',(-0.0717778861362653,-0.407041111792943,
-1.70562212620408));
#8304=CARTESIAN_POINT('Ctrl Pts',(-0.034424404517331,-0.411552957311693,
-1.706752));
#8305=CARTESIAN_POINT('Ctrl Pts',(0.0344244045173312,-0.411552957311693,
-1.706752));
#8306=CARTESIAN_POINT('Ctrl Pts',(0.0717778861362655,-0.407041111792943,
-1.70562212620408));
#8307=CARTESIAN_POINT('Ctrl Pts',(0.143648558862931,-0.387888272594439,
-1.70107730356824));
#8308=CARTESIAN_POINT('Ctrl Pts',(0.178166559972324,-0.373243761060364,
-1.69769003172132));
#8309=CARTESIAN_POINT('Ctrl Pts',(0.244262842368623,-0.335108247315849,
-1.68958170688653));
#8310=CARTESIAN_POINT('Ctrl Pts',(0.283214707341173,-0.303141259068212,
-1.68332504372461));
#8311=CARTESIAN_POINT('Ctrl Pts',(0.341837165343982,-0.236152929235937,
-1.67246562047521));
#8312=CARTESIAN_POINT('Ctrl Pts',(0.368536561654407,-0.192480977588835,
-1.66658649961961));
#8313=CARTESIAN_POINT('Ctrl Pts',(0.394174530911059,-0.123823518623745,
-1.66063136041479));
#8314=CARTESIAN_POINT('Ctrl Pts',(0.400393769631748,-0.101649918886749,
-1.65912839404491));
#8315=CARTESIAN_POINT('Ctrl Pts',(0.404717578595296,-0.0793800000000001,
-1.65807299932179));
#8316=CARTESIAN_POINT('',(0.886256117232623,-0.07938,-1.45861320581289));
#8317=CARTESIAN_POINT('Origin',(0.,-0.07938,0.));
#8318=CARTESIAN_POINT('',(1.45861320581289,-0.07938,-0.886256117232623));
#8319=CARTESIAN_POINT('Ctrl Pts',(0.886256117232623,-0.0793800000000001,
-1.45861320581289));
#8320=CARTESIAN_POINT('Ctrl Pts',(0.890059788636852,-0.101649918886749,
-1.45630208793976));
#8321=CARTESIAN_POINT('Ctrl Pts',(0.895520212222106,-0.123823518623745,
-1.45296717977858));
#8322=CARTESIAN_POINT('Ctrl Pts',(0.917859913453974,-0.192480977588835,
-1.43904931717599));
#8323=CARTESIAN_POINT('Ctrl Pts',(0.940896403863072,-0.236152929235937,
-1.4243271592157));
#8324=CARTESIAN_POINT('Ctrl Pts',(0.990027513266106,-0.303141259068211,
-1.39055359345152));
#8325=CARTESIAN_POINT('Ctrl Pts',(1.02199477007745,-0.335108247315849,-1.36743459453896));
#8326=CARTESIAN_POINT('Ctrl Pts',(1.07446535104584,-0.373243761060364,-1.32643091652006));
#8327=CARTESIAN_POINT('Ctrl Pts',(1.10126842659597,-0.387888272594439,-1.30441816675528));
#8328=CARTESIAN_POINT('Ctrl Pts',(1.15530234155453,-0.407041111792943,-1.25681160160691));
#8329=CARTESIAN_POINT('Ctrl Pts',(1.18251418313119,-0.411552957311693,-1.23119764287622));
#8330=CARTESIAN_POINT('Ctrl Pts',(1.23119764287622,-0.411552957311693,-1.18251418313119));
#8331=CARTESIAN_POINT('Ctrl Pts',(1.25681160160691,-0.407041111792943,-1.15530234155453));
#8332=CARTESIAN_POINT('Ctrl Pts',(1.30441816675528,-0.387888272594439,-1.10126842659597));
#8333=CARTESIAN_POINT('Ctrl Pts',(1.32643091652006,-0.373243761060364,-1.07446535104584));
#8334=CARTESIAN_POINT('Ctrl Pts',(1.36743459453896,-0.335108247315849,-1.02199477007745));
#8335=CARTESIAN_POINT('Ctrl Pts',(1.39055359345152,-0.303141259068212,-0.990027513266105));
#8336=CARTESIAN_POINT('Ctrl Pts',(1.4243271592157,-0.236152929235937,-0.940896403863071));
#8337=CARTESIAN_POINT('Ctrl Pts',(1.43904931717599,-0.192480977588835,-0.917859913453974));
#8338=CARTESIAN_POINT('Ctrl Pts',(1.45296717977858,-0.123823518623745,-0.895520212222106));
#8339=CARTESIAN_POINT('Ctrl Pts',(1.45630208793976,-0.101649918886749,-0.890059788636852));
#8340=CARTESIAN_POINT('Ctrl Pts',(1.45861320581289,-0.0793800000000001,
-0.886256117232623));
#8341=CARTESIAN_POINT('',(1.65807299932179,-0.07938,-0.404717578595296));
#8342=CARTESIAN_POINT('Origin',(0.,-0.07938,0.));
#8343=CARTESIAN_POINT('',(1.65807299932179,-0.07938,0.404717578595296));
#8344=CARTESIAN_POINT('Ctrl Pts',(1.65807299932179,-0.0793800000000001,
-0.404717578595296));
#8345=CARTESIAN_POINT('Ctrl Pts',(1.65912839404491,-0.101649918886749,-0.400393769631747));
#8346=CARTESIAN_POINT('Ctrl Pts',(1.66063136041479,-0.123823518623745,-0.394174530911058));
#8347=CARTESIAN_POINT('Ctrl Pts',(1.66658649961961,-0.192480977588835,-0.368536561654407));
#8348=CARTESIAN_POINT('Ctrl Pts',(1.67246562047521,-0.236152929235937,-0.341837165343982));
#8349=CARTESIAN_POINT('Ctrl Pts',(1.68332504372461,-0.303141259068212,-0.283214707341173));
#8350=CARTESIAN_POINT('Ctrl Pts',(1.68958170688653,-0.335108247315849,-0.244262842368623));
#8351=CARTESIAN_POINT('Ctrl Pts',(1.69769003172132,-0.373243761060364,-0.178166559972324));
#8352=CARTESIAN_POINT('Ctrl Pts',(1.70107730356824,-0.387888272594439,-0.143648558862931));
#8353=CARTESIAN_POINT('Ctrl Pts',(1.70562212620408,-0.407041111792943,-0.0717778861362655));
#8354=CARTESIAN_POINT('Ctrl Pts',(1.706752,-0.411552957311693,-0.0344244045173312));
#8355=CARTESIAN_POINT('Ctrl Pts',(1.706752,-0.411552957311693,0.0344244045173312));
#8356=CARTESIAN_POINT('Ctrl Pts',(1.70562212620408,-0.407041111792943,0.0717778861362655));
#8357=CARTESIAN_POINT('Ctrl Pts',(1.70107730356824,-0.387888272594439,0.143648558862931));
#8358=CARTESIAN_POINT('Ctrl Pts',(1.69769003172132,-0.373243761060364,0.178166559972324));
#8359=CARTESIAN_POINT('Ctrl Pts',(1.68958170688653,-0.335108247315849,0.244262842368623));
#8360=CARTESIAN_POINT('Ctrl Pts',(1.68332504372461,-0.303141259068212,0.283214707341173));
#8361=CARTESIAN_POINT('Ctrl Pts',(1.67246562047521,-0.236152929235937,0.341837165343982));
#8362=CARTESIAN_POINT('Ctrl Pts',(1.66658649961961,-0.192480977588835,0.368536561654407));
#8363=CARTESIAN_POINT('Ctrl Pts',(1.66063136041479,-0.123823518623745,0.394174530911058));
#8364=CARTESIAN_POINT('Ctrl Pts',(1.65912839404491,-0.101649918886749,0.400393769631747));
#8365=CARTESIAN_POINT('Ctrl Pts',(1.65807299932179,-0.0793800000000001,
0.404717578595296));
#8366=CARTESIAN_POINT('Origin',(0.,-0.07938,0.));
#8367=CARTESIAN_POINT('Origin',(0.,-0.07938,0.));
#8368=CARTESIAN_POINT('',(0.397005914195118,-0.07938,1.59456899932179));
#8369=CARTESIAN_POINT('Origin',(0.,-0.07938,0.));
#8370=CARTESIAN_POINT('Origin',(-3.33066907387547E-16,-0.07938,1.675));
#8371=CARTESIAN_POINT('Origin',(-3.33066907387547E-16,0.,1.675));
#8372=CARTESIAN_POINT('',(-0.397005914195118,-0.07938,1.59456899932179));
#8373=CARTESIAN_POINT('Ctrl Pts',(-0.397005914195119,-0.0793800000000001,
1.59456899932179));
#8374=CARTESIAN_POINT('Ctrl Pts',(-0.3886265584581,-0.123401821157026,1.59665523941937));
#8375=CARTESIAN_POINT('Ctrl Pts',(-0.373030350867485,-0.166543350814306,
1.60050712143809));
#8376=CARTESIAN_POINT('Ctrl Pts',(-0.333298652394954,-0.237231147975234,
1.60919314384089));
#8377=CARTESIAN_POINT('Ctrl Pts',(-0.311480544243687,-0.266264900654909,
1.61365775139403));
#8378=CARTESIAN_POINT('Ctrl Pts',(-0.261368388670537,-0.317195968905306,
1.62252828437015));
#8379=CARTESIAN_POINT('Ctrl Pts',(-0.233069203882014,-0.33909093068465,
1.62691869420078));
#8380=CARTESIAN_POINT('Ctrl Pts',(-0.174042761838764,-0.373586846396559,
1.63426473152765));
#8381=CARTESIAN_POINT('Ctrl Pts',(-0.14036578147155,-0.388086240756494,
1.63761964365402));
#8382=CARTESIAN_POINT('Ctrl Pts',(-0.0701778381840615,-0.407068917407805,
1.64212536811722));
#8383=CARTESIAN_POINT('Ctrl Pts',(-0.0336652739555918,-0.411552957311693,
1.643248));
#8384=CARTESIAN_POINT('Ctrl Pts',(0.0336652739555913,-0.411552957311693,
1.643248));
#8385=CARTESIAN_POINT('Ctrl Pts',(0.070177838184061,-0.407068917407805,
1.64212536811722));
#8386=CARTESIAN_POINT('Ctrl Pts',(0.140365781471549,-0.388086240756494,
1.63761964365402));
#8387=CARTESIAN_POINT('Ctrl Pts',(0.174042761838763,-0.373586846396559,
1.63426473152765));
#8388=CARTESIAN_POINT('Ctrl Pts',(0.233069203882014,-0.33909093068465,1.62691869420078));
#8389=CARTESIAN_POINT('Ctrl Pts',(0.261368388670536,-0.317195968905306,
1.62252828437015));
#8390=CARTESIAN_POINT('Ctrl Pts',(0.311480544243686,-0.266264900654908,
1.61365775139403));
#8391=CARTESIAN_POINT('Ctrl Pts',(0.333298652394954,-0.237231147975234,
1.60919314384089));
#8392=CARTESIAN_POINT('Ctrl Pts',(0.373030350867484,-0.166543350814306,
1.60050712143809));
#8393=CARTESIAN_POINT('Ctrl Pts',(0.388626558458099,-0.123401821157026,
1.59665523941937));
#8394=CARTESIAN_POINT('Ctrl Pts',(0.397005914195118,-0.07938,1.59456899932179));
#8395=CARTESIAN_POINT('Origin',(-3.33066907387547E-16,-0.07938,1.675));
#8396=CARTESIAN_POINT('Origin',(0.,-0.07938,0.));
#8397=CARTESIAN_POINT('',(-0.846804978391754,-0.07938,1.40825612658882));
#8398=CARTESIAN_POINT('Origin',(0.,-0.07938,0.));
#8399=CARTESIAN_POINT('Origin',(-1.18440385848747,-0.07938,1.18440385848747));
#8400=CARTESIAN_POINT('Origin',(-1.18440385848747,0.,1.18440385848747));
#8401=CARTESIAN_POINT('',(-1.40825612658882,-0.07938,0.846804978391753));
#8402=CARTESIAN_POINT('Ctrl Pts',(-1.40825612658882,-0.0793800000000001,
0.846804978391753));
#8403=CARTESIAN_POINT('Ctrl Pts',(-1.40380622184538,-0.123401821157026,
0.854205272175555));
#8404=CARTESIAN_POINT('Ctrl Pts',(-1.39550172959303,-0.166543350814306,
0.867957148219442));
#8405=CARTESIAN_POINT('Ctrl Pts',(-1.3735491215176,-0.237231147975235,0.902193646979983));
#8406=CARTESIAN_POINT('Ctrl Pts',(-1.36127834356734,-0.266264900654909,
0.920778333482565));
#8407=CARTESIAN_POINT('Ctrl Pts',(-1.33211611256184,-0.317195968905306,
0.962485392528369));
#8408=CARTESIAN_POINT('Ctrl Pts',(-1.31521005565926,-0.339090930684651,
0.985600426557816));
#8409=CARTESIAN_POINT('Ctrl Pts',(-1.27866649102984,-0.373586846396559,
1.03253285680459));
#8410=CARTESIAN_POINT('Ctrl Pts',(-1.25722555095714,-0.388086240756494,
1.05871835910697));
#8411=CARTESIAN_POINT('Ctrl Pts',(-1.2107812086231,-0.407068917407805,1.11153475808518));
#8412=CARTESIAN_POINT('Ctrl Pts',(-1.18575674747573,-0.411552957311693,
1.13814686046673));
#8413=CARTESIAN_POINT('Ctrl Pts',(-1.13814686046673,-0.411552957311693,
1.18575674747573));
#8414=CARTESIAN_POINT('Ctrl Pts',(-1.11153475808518,-0.407068917407805,
1.2107812086231));
#8415=CARTESIAN_POINT('Ctrl Pts',(-1.05871835910697,-0.388086240756494,
1.25722555095714));
#8416=CARTESIAN_POINT('Ctrl Pts',(-1.03253285680459,-0.373586846396559,
1.27866649102984));
#8417=CARTESIAN_POINT('Ctrl Pts',(-0.985600426557816,-0.33909093068465,
1.31521005565926));
#8418=CARTESIAN_POINT('Ctrl Pts',(-0.962485392528369,-0.317195968905306,
1.33211611256184));
#8419=CARTESIAN_POINT('Ctrl Pts',(-0.920778333482565,-0.266264900654908,
1.36127834356734));
#8420=CARTESIAN_POINT('Ctrl Pts',(-0.902193646979983,-0.237231147975234,
1.3735491215176));
#8421=CARTESIAN_POINT('Ctrl Pts',(-0.867957148219442,-0.166543350814306,
1.39550172959303));
#8422=CARTESIAN_POINT('Ctrl Pts',(-0.854205272175555,-0.123401821157026,
1.40380622184538));
#8423=CARTESIAN_POINT('Ctrl Pts',(-0.846804978391753,-0.0793800000000001,
1.40825612658882));
#8424=CARTESIAN_POINT('Origin',(-1.18440385848747,-0.07938,1.18440385848747));
#8425=CARTESIAN_POINT('Origin',(0.,-0.07938,0.));
#8426=CARTESIAN_POINT('',(-1.59456899932179,-0.07938,0.397005914195118));
#8427=CARTESIAN_POINT('Origin',(0.,-0.07938,0.));
#8428=CARTESIAN_POINT('Origin',(-1.675,-0.07938,-2.22044604925031E-16));
#8429=CARTESIAN_POINT('Origin',(-1.675,0.,-2.22044604925031E-16));
#8430=CARTESIAN_POINT('',(-1.59456899932179,-0.07938,-0.397005914195118));
#8431=CARTESIAN_POINT('',(-1.643248,-0.411552957311693,3.47540551556327E-18));
#8432=CARTESIAN_POINT('Ctrl Pts',(-1.59456899932179,-0.0793800000000001,
-0.397005914195119));
#8433=CARTESIAN_POINT('Ctrl Pts',(-1.59665523941937,-0.123401821157026,
-0.388626558458099));
#8434=CARTESIAN_POINT('Ctrl Pts',(-1.60050712143809,-0.166543350814306,
-0.373030350867485));
#8435=CARTESIAN_POINT('Ctrl Pts',(-1.60919314384089,-0.237231147975234,
-0.333298652394954));
#8436=CARTESIAN_POINT('Ctrl Pts',(-1.61365775139403,-0.266264900654909,
-0.311480544243686));
#8437=CARTESIAN_POINT('Ctrl Pts',(-1.62252828437015,-0.317195968905306,
-0.261368388670537));
#8438=CARTESIAN_POINT('Ctrl Pts',(-1.62691869420078,-0.33909093068465,-0.233069203882014));
#8439=CARTESIAN_POINT('Ctrl Pts',(-1.63426473152765,-0.373586846396559,
-0.174042761838764));
#8440=CARTESIAN_POINT('Ctrl Pts',(-1.63761964365402,-0.388086240756494,
-0.140365781471549));
#8441=CARTESIAN_POINT('Ctrl Pts',(-1.64212536811722,-0.407068917407805,
-0.0701778381840614));
#8442=CARTESIAN_POINT('Ctrl Pts',(-1.643248,-0.411552957311693,-0.0336652739555917));
#8443=CARTESIAN_POINT('Ctrl Pts',(-1.643248,-0.411552957311693,-2.0122792321331E-16));
#8444=CARTESIAN_POINT('Origin',(-1.675,-0.07938,-2.22044604925031E-16));
#8445=CARTESIAN_POINT('Ctrl Pts',(-1.643248,-0.411552957311693,-1.94289029309402E-16));
#8446=CARTESIAN_POINT('Ctrl Pts',(-1.643248,-0.411552957311693,0.0336652739555913));
#8447=CARTESIAN_POINT('Ctrl Pts',(-1.64212536811722,-0.407068917407805,
0.0701778381840609));
#8448=CARTESIAN_POINT('Ctrl Pts',(-1.63761964365402,-0.388086240756494,
0.140365781471549));
#8449=CARTESIAN_POINT('Ctrl Pts',(-1.63426473152765,-0.373586846396559,
0.174042761838763));
#8450=CARTESIAN_POINT('Ctrl Pts',(-1.62691869420078,-0.33909093068465,0.233069203882014));
#8451=CARTESIAN_POINT('Ctrl Pts',(-1.62252828437015,-0.317195968905306,
0.261368388670536));
#8452=CARTESIAN_POINT('Ctrl Pts',(-1.61365775139403,-0.266264900654909,
0.311480544243686));
#8453=CARTESIAN_POINT('Ctrl Pts',(-1.60919314384089,-0.237231147975235,
0.333298652394954));
#8454=CARTESIAN_POINT('Ctrl Pts',(-1.60050712143809,-0.166543350814306,
0.373030350867484));
#8455=CARTESIAN_POINT('Ctrl Pts',(-1.59665523941937,-0.123401821157026,
0.388626558458099));
#8456=CARTESIAN_POINT('Ctrl Pts',(-1.59456899932179,-0.0793800000000001,
0.397005914195118));
#8457=CARTESIAN_POINT('Origin',(0.,-0.07938,0.));
#8458=CARTESIAN_POINT('',(-1.40825612658882,-0.07938,-0.846804978391753));
#8459=CARTESIAN_POINT('Origin',(0.,-0.07938,0.));
#8460=CARTESIAN_POINT('Origin',(-1.18440385848747,-0.07938,-1.18440385848747));
#8461=CARTESIAN_POINT('Origin',(-1.18440385848747,0.,-1.18440385848747));
#8462=CARTESIAN_POINT('',(-0.846804978391753,-0.07938,-1.40825612658882));
#8463=CARTESIAN_POINT('Ctrl Pts',(-0.846804978391753,-0.0793800000000001,
-1.40825612658882));
#8464=CARTESIAN_POINT('Ctrl Pts',(-0.854205272175555,-0.123401821157026,
-1.40380622184538));
#8465=CARTESIAN_POINT('Ctrl Pts',(-0.867957148219442,-0.166543350814306,
-1.39550172959303));
#8466=CARTESIAN_POINT('Ctrl Pts',(-0.902193646979982,-0.237231147975234,
-1.3735491215176));
#8467=CARTESIAN_POINT('Ctrl Pts',(-0.920778333482564,-0.266264900654908,
-1.36127834356734));
#8468=CARTESIAN_POINT('Ctrl Pts',(-0.962485392528368,-0.317195968905306,
-1.33211611256184));
#8469=CARTESIAN_POINT('Ctrl Pts',(-0.985600426557816,-0.33909093068465,
-1.31521005565926));
#8470=CARTESIAN_POINT('Ctrl Pts',(-1.03253285680459,-0.373586846396559,
-1.27866649102984));
#8471=CARTESIAN_POINT('Ctrl Pts',(-1.05871835910697,-0.388086240756494,
-1.25722555095714));
#8472=CARTESIAN_POINT('Ctrl Pts',(-1.11153475808518,-0.407068917407805,
-1.2107812086231));
#8473=CARTESIAN_POINT('Ctrl Pts',(-1.13814686046673,-0.411552957311693,
-1.18575674747573));
#8474=CARTESIAN_POINT('Ctrl Pts',(-1.18575674747573,-0.411552957311693,
-1.13814686046673));
#8475=CARTESIAN_POINT('Ctrl Pts',(-1.2107812086231,-0.407068917407805,-1.11153475808518));
#8476=CARTESIAN_POINT('Ctrl Pts',(-1.25722555095714,-0.388086240756494,
-1.05871835910697));
#8477=CARTESIAN_POINT('Ctrl Pts',(-1.27866649102984,-0.373586846396559,
-1.03253285680459));
#8478=CARTESIAN_POINT('Ctrl Pts',(-1.31521005565926,-0.33909093068465,-0.985600426557816));
#8479=CARTESIAN_POINT('Ctrl Pts',(-1.33211611256184,-0.317195968905306,
-0.962485392528369));
#8480=CARTESIAN_POINT('Ctrl Pts',(-1.36127834356734,-0.266264900654909,
-0.920778333482565));
#8481=CARTESIAN_POINT('Ctrl Pts',(-1.3735491215176,-0.237231147975234,-0.902193646979983));
#8482=CARTESIAN_POINT('Ctrl Pts',(-1.39550172959303,-0.166543350814306,
-0.867957148219442));
#8483=CARTESIAN_POINT('Ctrl Pts',(-1.40380622184538,-0.123401821157026,
-0.854205272175555));
#8484=CARTESIAN_POINT('Ctrl Pts',(-1.40825612658882,-0.07938,-0.846804978391753));
#8485=CARTESIAN_POINT('Origin',(-1.18440385848747,-0.07938,-1.18440385848747));
#8486=CARTESIAN_POINT('Origin',(0.,-0.07938,0.));
#8487=CARTESIAN_POINT('',(-0.397005914195118,-0.07938,-1.59456899932179));
#8488=CARTESIAN_POINT('Origin',(0.,-0.07938,0.));
#8489=CARTESIAN_POINT('Origin',(1.11022302462516E-16,-0.07938,-1.675));
#8490=CARTESIAN_POINT('Origin',(1.11022302462516E-16,0.,-1.675));
#8491=CARTESIAN_POINT('',(0.397005914195118,-0.07938,-1.59456899932179));
#8492=CARTESIAN_POINT('Ctrl Pts',(0.397005914195119,-0.0793800000000001,
-1.59456899932179));
#8493=CARTESIAN_POINT('Ctrl Pts',(0.388626558458099,-0.123401821157026,
-1.59665523941937));
#8494=CARTESIAN_POINT('Ctrl Pts',(0.373030350867485,-0.166543350814306,
-1.60050712143809));
#8495=CARTESIAN_POINT('Ctrl Pts',(0.333298652394954,-0.237231147975234,
-1.60919314384089));
#8496=CARTESIAN_POINT('Ctrl Pts',(0.311480544243686,-0.266264900654909,
-1.61365775139403));
#8497=CARTESIAN_POINT('Ctrl Pts',(0.261368388670537,-0.317195968905306,
-1.62252828437015));
#8498=CARTESIAN_POINT('Ctrl Pts',(0.233069203882014,-0.33909093068465,-1.62691869420078));
#8499=CARTESIAN_POINT('Ctrl Pts',(0.174042761838763,-0.373586846396559,
-1.63426473152765));
#8500=CARTESIAN_POINT('Ctrl Pts',(0.140365781471549,-0.388086240756494,
-1.63761964365402));
#8501=CARTESIAN_POINT('Ctrl Pts',(0.0701778381840612,-0.407068917407805,
-1.64212536811722));
#8502=CARTESIAN_POINT('Ctrl Pts',(0.0336652739555916,-0.411552957311693,
-1.643248));
#8503=CARTESIAN_POINT('Ctrl Pts',(-0.0336652739555915,-0.411552957311693,
-1.643248));
#8504=CARTESIAN_POINT('Ctrl Pts',(-0.0701778381840612,-0.407068917407805,
-1.64212536811722));
#8505=CARTESIAN_POINT('Ctrl Pts',(-0.140365781471549,-0.388086240756494,
-1.63761964365402));
#8506=CARTESIAN_POINT('Ctrl Pts',(-0.174042761838764,-0.373586846396559,
-1.63426473152765));
#8507=CARTESIAN_POINT('Ctrl Pts',(-0.233069203882014,-0.33909093068465,
-1.62691869420078));
#8508=CARTESIAN_POINT('Ctrl Pts',(-0.261368388670536,-0.317195968905306,
-1.62252828437015));
#8509=CARTESIAN_POINT('Ctrl Pts',(-0.311480544243686,-0.266264900654908,
-1.61365775139403));
#8510=CARTESIAN_POINT('Ctrl Pts',(-0.333298652394954,-0.237231147975234,
-1.60919314384089));
#8511=CARTESIAN_POINT('Ctrl Pts',(-0.373030350867485,-0.166543350814306,
-1.60050712143809));
#8512=CARTESIAN_POINT('Ctrl Pts',(-0.388626558458099,-0.123401821157026,
-1.59665523941937));
#8513=CARTESIAN_POINT('Ctrl Pts',(-0.397005914195118,-0.07938,-1.59456899932179));
#8514=CARTESIAN_POINT('Origin',(1.11022302462516E-16,-0.07938,-1.675));
#8515=CARTESIAN_POINT('Origin',(0.,-0.07938,0.));
#8516=CARTESIAN_POINT('',(0.846804978391753,-0.07938,-1.40825612658882));
#8517=CARTESIAN_POINT('Origin',(0.,-0.07938,0.));
#8518=CARTESIAN_POINT('Origin',(1.18440385848747,-0.07938,-1.18440385848747));
#8519=CARTESIAN_POINT('Origin',(1.18440385848747,0.,-1.18440385848747));
#8520=CARTESIAN_POINT('',(1.40825612658882,-0.07938,-0.846804978391753));
#8521=CARTESIAN_POINT('Ctrl Pts',(1.40825612658882,-0.0793800000000001,
-0.846804978391753));
#8522=CARTESIAN_POINT('Ctrl Pts',(1.40380622184538,-0.123401821157026,-0.854205272175555));
#8523=CARTESIAN_POINT('Ctrl Pts',(1.39550172959303,-0.166543350814306,-0.867957148219442));
#8524=CARTESIAN_POINT('Ctrl Pts',(1.3735491215176,-0.237231147975234,-0.902193646979983));
#8525=CARTESIAN_POINT('Ctrl Pts',(1.36127834356734,-0.266264900654908,-0.920778333482565));
#8526=CARTESIAN_POINT('Ctrl Pts',(1.33211611256184,-0.317195968905306,-0.962485392528369));
#8527=CARTESIAN_POINT('Ctrl Pts',(1.31521005565926,-0.33909093068465,-0.985600426557816));
#8528=CARTESIAN_POINT('Ctrl Pts',(1.27866649102984,-0.373586846396559,-1.03253285680459));
#8529=CARTESIAN_POINT('Ctrl Pts',(1.25722555095714,-0.388086240756494,-1.05871835910697));
#8530=CARTESIAN_POINT('Ctrl Pts',(1.2107812086231,-0.407068917407805,-1.11153475808518));
#8531=CARTESIAN_POINT('Ctrl Pts',(1.18575674747573,-0.411552957311693,-1.13814686046673));
#8532=CARTESIAN_POINT('Ctrl Pts',(1.13814686046673,-0.411552957311693,-1.18575674747573));
#8533=CARTESIAN_POINT('Ctrl Pts',(1.11153475808518,-0.407068917407805,-1.2107812086231));
#8534=CARTESIAN_POINT('Ctrl Pts',(1.05871835910697,-0.388086240756494,-1.25722555095714));
#8535=CARTESIAN_POINT('Ctrl Pts',(1.03253285680459,-0.373586846396559,-1.27866649102984));
#8536=CARTESIAN_POINT('Ctrl Pts',(0.985600426557816,-0.33909093068465,-1.31521005565926));
#8537=CARTESIAN_POINT('Ctrl Pts',(0.962485392528369,-0.317195968905306,
-1.33211611256184));
#8538=CARTESIAN_POINT('Ctrl Pts',(0.920778333482565,-0.266264900654909,
-1.36127834356734));
#8539=CARTESIAN_POINT('Ctrl Pts',(0.902193646979983,-0.237231147975234,
-1.3735491215176));
#8540=CARTESIAN_POINT('Ctrl Pts',(0.867957148219442,-0.166543350814306,
-1.39550172959303));
#8541=CARTESIAN_POINT('Ctrl Pts',(0.854205272175555,-0.123401821157026,
-1.40380622184538));
#8542=CARTESIAN_POINT('Ctrl Pts',(0.846804978391753,-0.0793800000000001,
-1.40825612658882));
#8543=CARTESIAN_POINT('Origin',(1.18440385848747,-0.07938,-1.18440385848747));
#8544=CARTESIAN_POINT('Origin',(0.,-0.27783,0.));
#8545=CARTESIAN_POINT('',(-1.643248,-0.47628,2.01239840340529E-16));
#8546=CARTESIAN_POINT('Origin',(0.,-0.47628,0.));
#8547=CARTESIAN_POINT('',(-1.643248,-0.27783,2.01239840340529E-16));
#8548=CARTESIAN_POINT('',(1.59456899932179,-0.07938,0.397005914195118));
#8549=CARTESIAN_POINT('Origin',(0.,-0.07938,0.));
#8550=CARTESIAN_POINT('',(1.59456899932179,-0.07938,-0.397005914195118));
#8551=CARTESIAN_POINT('Ctrl Pts',(1.59456899932179,-0.0793800000000001,
0.397005914195118));
#8552=CARTESIAN_POINT('Ctrl Pts',(1.59665523941937,-0.123401821157026,0.388626558458099));
#8553=CARTESIAN_POINT('Ctrl Pts',(1.60050712143809,-0.166543350814306,0.373030350867485));
#8554=CARTESIAN_POINT('Ctrl Pts',(1.60919314384089,-0.237231147975234,0.333298652394954));
#8555=CARTESIAN_POINT('Ctrl Pts',(1.61365775139403,-0.266264900654909,0.311480544243686));
#8556=CARTESIAN_POINT('Ctrl Pts',(1.62252828437015,-0.317195968905306,0.261368388670537));
#8557=CARTESIAN_POINT('Ctrl Pts',(1.62691869420078,-0.33909093068465,0.233069203882014));
#8558=CARTESIAN_POINT('Ctrl Pts',(1.63426473152765,-0.373586846396559,0.174042761838764));
#8559=CARTESIAN_POINT('Ctrl Pts',(1.63761964365402,-0.388086240756494,0.140365781471549));
#8560=CARTESIAN_POINT('Ctrl Pts',(1.64212536811722,-0.407068917407805,0.0701778381840612));
#8561=CARTESIAN_POINT('Ctrl Pts',(1.643248,-0.411552957311693,0.0336652739555916));
#8562=CARTESIAN_POINT('Ctrl Pts',(1.643248,-0.411552957311693,-0.0336652739555916));
#8563=CARTESIAN_POINT('Ctrl Pts',(1.64212536811722,-0.407068917407805,-0.0701778381840612));
#8564=CARTESIAN_POINT('Ctrl Pts',(1.63761964365402,-0.388086240756494,-0.140365781471549));
#8565=CARTESIAN_POINT('Ctrl Pts',(1.63426473152765,-0.373586846396559,-0.174042761838764));
#8566=CARTESIAN_POINT('Ctrl Pts',(1.62691869420078,-0.33909093068465,-0.233069203882014));
#8567=CARTESIAN_POINT('Ctrl Pts',(1.62252828437015,-0.317195968905306,-0.261368388670537));
#8568=CARTESIAN_POINT('Ctrl Pts',(1.61365775139403,-0.266264900654909,-0.311480544243686));
#8569=CARTESIAN_POINT('Ctrl Pts',(1.60919314384089,-0.237231147975234,-0.333298652394954));
#8570=CARTESIAN_POINT('Ctrl Pts',(1.60050712143809,-0.166543350814306,-0.373030350867485));
#8571=CARTESIAN_POINT('Ctrl Pts',(1.59665523941937,-0.123401821157026,-0.388626558458099));
#8572=CARTESIAN_POINT('Ctrl Pts',(1.59456899932179,-0.07938,-0.397005914195118));
#8573=CARTESIAN_POINT('Origin',(0.,-0.07938,0.));
#8574=CARTESIAN_POINT('Origin',(0.,-0.07938,0.));
#8575=CARTESIAN_POINT('Origin',(1.675,-0.07938,0.));
#8576=CARTESIAN_POINT('Origin',(1.675,0.,0.));
#8577=CARTESIAN_POINT('Origin',(1.675,-0.07938,0.));
#8578=CARTESIAN_POINT('Origin',(0.,-0.47628,0.));
#8579=CARTESIAN_POINT('Origin',(0.,-0.07938,0.));
#9402=UNCERTAINTY_MEASURE_WITH_UNIT(LENGTH_MEASURE(0.001),#9449,
'DISTANCE_ACCURACY_VALUE',
'Maximum model space distance between geometric entities at asserted c
onnectivities');
#9416=UNCERTAINTY_MEASURE_WITH_UNIT(LENGTH_MEASURE(0.001),#9449,
'DISTANCE_ACCURACY_VALUE',
'Maximum model space distance between geometric entities at asserted c
onnectivities');
#9434=(
GEOMETRIC_REPRESENTATION_CONTEXT(3)
GLOBAL_UNCERTAINTY_ASSIGNED_CONTEXT((#9402))
GLOBAL_UNIT_ASSIGNED_CONTEXT((#9449,#9451,#9452))
REPRESENTATION_CONTEXT('','3D')
);
#9448=(
GEOMETRIC_REPRESENTATION_CONTEXT(3)
GLOBAL_UNCERTAINTY_ASSIGNED_CONTEXT((#9416))
GLOBAL_UNIT_ASSIGNED_CONTEXT((#9449,#9451,#9452))
REPRESENTATION_CONTEXT('','3D')
);
#9449=(
LENGTH_UNIT()
NAMED_UNIT(*)
SI_UNIT(.CENTI.,.METRE.)
);
#9451=(
NAMED_UNIT(*)
PLANE_ANGLE_UNIT()
SI_UNIT($,.RADIAN.)
);
#9452=(
NAMED_UNIT(*)
SI_UNIT($,.STERADIAN.)
SOLID_ANGLE_UNIT()
);
#9470=SHAPE_DEFINITION_REPRESENTATION(#9501,#9574);
#9501=PRODUCT_DEFINITION_SHAPE('',$,#9606);
#9574=SHAPE_REPRESENTATION('',(#5485),#9434);
#9588=PRODUCT_DEFINITION_CONTEXT('part definition',#9683,'design');
#9606=PRODUCT_DEFINITION('Cage','Cage',#9637,#9588);
#9637=PRODUCT_DEFINITION_FORMATION('',$,#9702);
#9683=APPLICATION_CONTEXT(
'Core Data for Automotive Mechanical Design Process');
#9684=PRODUCT_CONTEXT('part definition',#9683,'mechanical');
#9702=PRODUCT('Cage','Cage','Cage',(#9684));
#9772=COLOUR_RGB('Grey',0.48,0.52,0.57);
#9773=FILL_AREA_STYLE_COLOUR('',#9772);
#9774=FILL_AREA_STYLE('',(#9773));
#9775=SURFACE_STYLE_FILL_AREA(#9774);
#9776=SURFACE_SIDE_STYLE('',(#9775));
#9777=SURFACE_STYLE_USAGE(.BOTH.,#9776);
#9778=PRESENTATION_STYLE_ASSIGNMENT((#9777));
ENDSEC;
END-ISO-10303-21;
